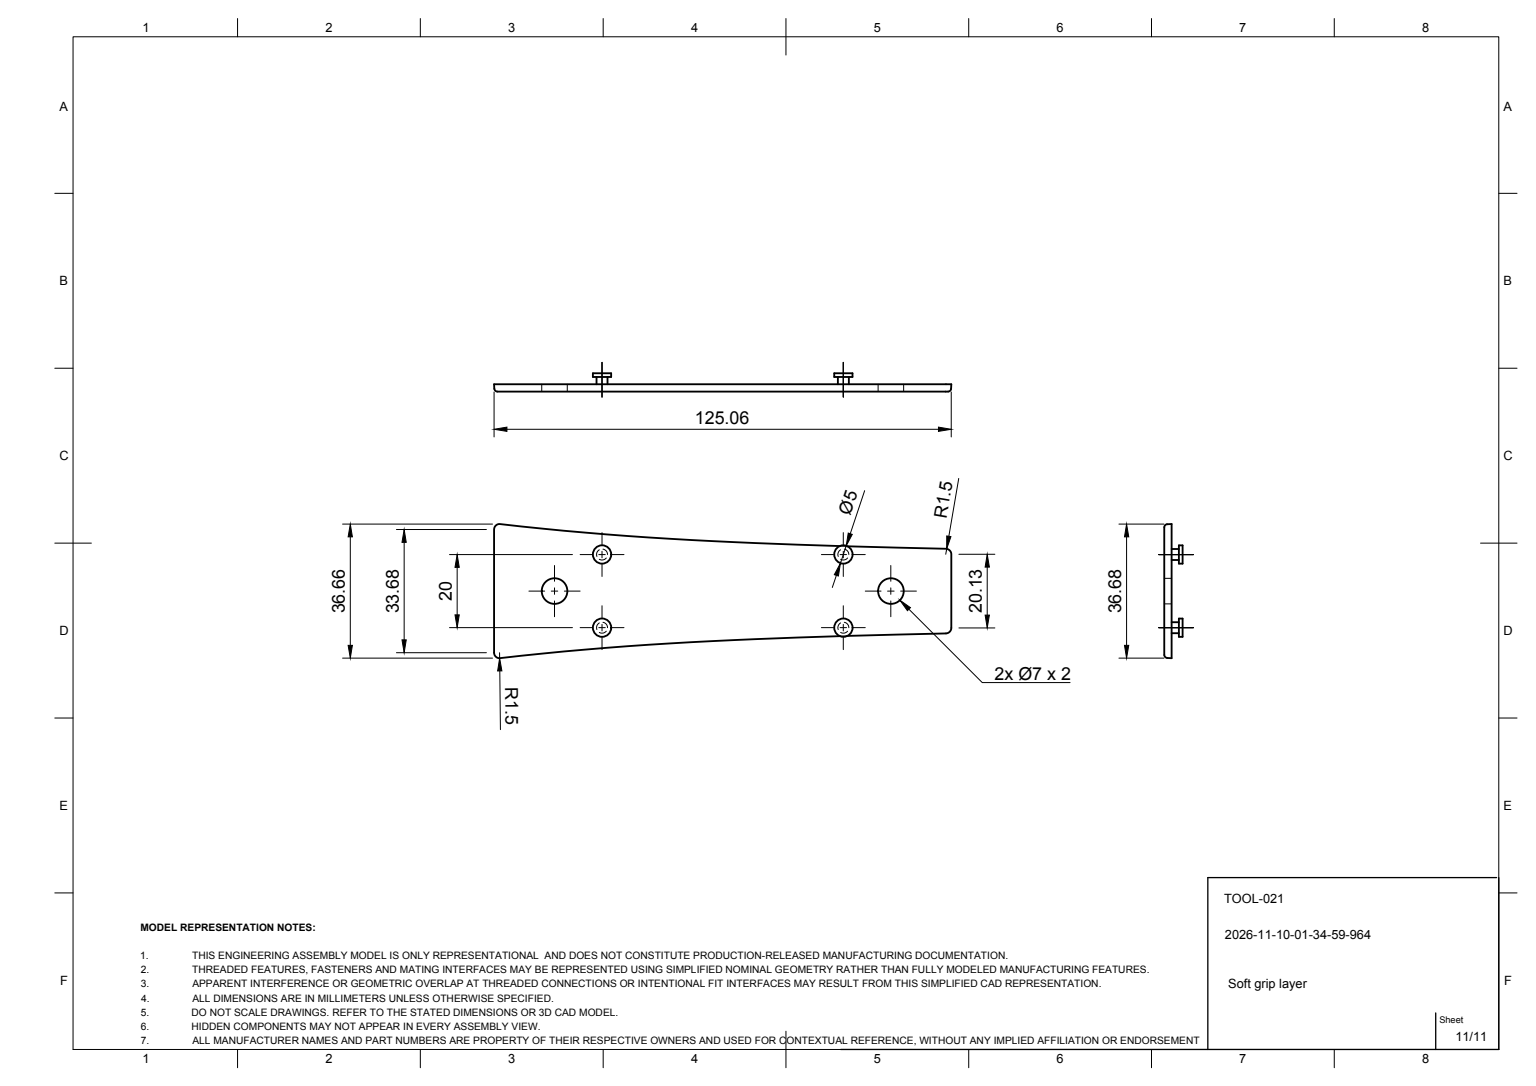
ISO-10303-21;
HEADER;
/* Generated by software containing ST-Developer
 * from STEP Tools, Inc. (www.steptools.com) 
 */

FILE_DESCRIPTION(
/* description */ (''),
/* implementation_level */ '2;1');

FILE_NAME(
/* name */ 'Soft grip layer.step',
/* time_stamp */ '2026-11-10T09:05:57-08:00',
/* author */ (''),
/* organization */ (''),
/* preprocessor_version */ 'ST-DEVELOPER v20.2',
/* originating_system */ 'Autodesk Translation Framework v15.17.0.0',
/* authorisation */ '');

FILE_SCHEMA (('AUTOMOTIVE_DESIGN { 1 0 10303 214 3 1 1 }'));
ENDSEC;

DATA;
#10=MECHANICAL_DESIGN_GEOMETRIC_PRESENTATION_REPRESENTATION('',(#571),#19618);
#155=B_SPLINE_SURFACE_WITH_KNOTS('',3,3,((#13946,#13947,#13948,#13949,#13950),
(#13951,#13952,#13953,#13954,#13955),(#13956,#13957,#13958,#13959,#13960),
(#13961,#13962,#13963,#13964,#13965),(#13966,#13967,#13968,#13969,#13970)),
 .UNSPECIFIED.,.F.,.F.,.F.,(4,1,4),(4,1,4),(0.,0.571428571428571,1.),(0.,
0.0505788685273923,0.118017359897249),.UNSPECIFIED.);
#156=B_SPLINE_SURFACE_WITH_KNOTS('',3,3,((#13993,#13994,#13995,#13996,#13997),
(#13998,#13999,#14000,#14001,#14002),(#14003,#14004,#14005,#14006,#14007),
(#14008,#14009,#14010,#14011,#14012),(#14013,#14014,#14015,#14016,#14017)),
 .UNSPECIFIED.,.F.,.F.,.F.,(4,1,4),(4,1,4),(0.,0.571428571428571,1.),(0.,
0.0505788685278266,0.118017359898262),.UNSPECIFIED.);
#157=B_SPLINE_SURFACE_WITH_KNOTS('',3,3,((#14031,#14032,#14033,#14034,#14035),
(#14036,#14037,#14038,#14039,#14040),(#14041,#14042,#14043,#14044,#14045),
(#14046,#14047,#14048,#14049,#14050),(#14051,#14052,#14053,#14054,#14055)),
 .UNSPECIFIED.,.F.,.F.,.F.,(4,1,4),(4,1,4),(0.,0.571428571428571,1.),(0.,
5.23288834931112,12.2100728150593),.UNSPECIFIED.);
#158=B_SPLINE_SURFACE_WITH_KNOTS('',3,3,((#14069,#14070,#14071,#14072,#14073),
(#14074,#14075,#14076,#14077,#14078),(#14079,#14080,#14081,#14082,#14083),
(#14084,#14085,#14086,#14087,#14088),(#14089,#14090,#14091,#14092,#14093)),
 .UNSPECIFIED.,.F.,.F.,.F.,(4,1,4),(4,1,4),(0.,0.571428571428571,1.),(1.97133828064127E-11,
0.0463413823988794,0.108129892237767),.UNSPECIFIED.);
#159=B_SPLINE_SURFACE_WITH_KNOTS('',3,3,((#14113,#14114,#14115,#14116,#14117),
(#14118,#14119,#14120,#14121,#14122),(#14123,#14124,#14125,#14126,#14127),
(#14128,#14129,#14130,#14131,#14132),(#14133,#14134,#14135,#14136,#14137)),
 .UNSPECIFIED.,.F.,.F.,.F.,(4,1,4),(4,1,4),(0.,0.571428571428571,1.),(0.,
0.0463413823743492,0.108129892206815),.UNSPECIFIED.);
#160=B_SPLINE_SURFACE_WITH_KNOTS('',3,3,((#14151,#14152,#14153,#14154,#14155),
(#14156,#14157,#14158,#14159,#14160),(#14161,#14162,#14163,#14164,#14165),
(#14166,#14167,#14168,#14169,#14170),(#14171,#14172,#14173,#14174,#14175)),
 .UNSPECIFIED.,.F.,.F.,.F.,(4,1,4),(4,1,4),(0.,0.571428571428571,1.),(6.51086303075479E-13,
6.97718480957529,12.2100734167563),.UNSPECIFIED.);
#161=B_SPLINE_SURFACE_WITH_KNOTS('',3,3,((#14198,#14199,#14200,#14201),
(#14202,#14203,#14204,#14205),(#14206,#14207,#14208,#14209),(#14210,#14211,
#14212,#14213),(#14214,#14215,#14216,#14217)),.UNSPECIFIED.,.F.,.F.,.F.,
(4,1,4),(4,4),(0.,0.571428571428571,1.),(-0.00308447593286339,0.124708996845866),
 .UNSPECIFIED.);
#162=B_SPLINE_SURFACE_WITH_KNOTS('',3,3,((#14251,#14252,#14253,#14254),
(#14255,#14256,#14257,#14258),(#14259,#14260,#14261,#14262),(#14263,#14264,
#14265,#14266)),.UNSPECIFIED.,.F.,.F.,.F.,(4,4),(4,4),(0.0116899650356219,
0.986620910196183),(0.,0.621418053543664),.UNSPECIFIED.);
#163=B_SPLINE_SURFACE_WITH_KNOTS('',3,3,((#14276,#14277,#14278,#14279),
(#14280,#14281,#14282,#14283),(#14284,#14285,#14286,#14287),(#14288,#14289,
#14290,#14291),(#14292,#14293,#14294,#14295),(#14296,#14297,#14298,#14299)),
 .UNSPECIFIED.,.F.,.F.,.F.,(4,1,1,4),(4,4),(0.,0.285714285714286,0.571428571428571,
1.),(-0.00421817271916687,0.124025126494243),.UNSPECIFIED.);
#164=B_SPLINE_SURFACE_WITH_KNOTS('',3,3,((#14347,#14348,#14349,#14350),
(#14351,#14352,#14353,#14354),(#14355,#14356,#14357,#14358),(#14359,#14360,
#14361,#14362),(#14363,#14364,#14365,#14366)),.UNSPECIFIED.,.F.,.F.,.F.,
(4,1,4),(4,4),(0.,0.571428571428571,1.),(-0.00306862226109154,0.124708996851356),
 .UNSPECIFIED.);
#165=B_SPLINE_SURFACE_WITH_KNOTS('',3,3,((#14400,#14401,#14402,#14403),
(#14404,#14405,#14406,#14407),(#14408,#14409,#14410,#14411),(#14412,#14413,
#14414,#14415),(#14416,#14417,#14418,#14419),(#14420,#14421,#14422,#14423)),
 .UNSPECIFIED.,.F.,.F.,.F.,(4,1,1,4),(4,4),(0.,0.285714285714286,0.571428571428571,
1.),(-0.00430078538920315,0.12402512649425),.UNSPECIFIED.);
#166=B_SPLINE_SURFACE_WITH_KNOTS('',3,3,((#14468,#14469,#14470,#14471),
(#14472,#14473,#14474,#14475),(#14476,#14477,#14478,#14479),(#14480,#14481,
#14482,#14483)),.UNSPECIFIED.,.F.,.F.,.F.,(4,4),(4,4),(0.0133790898038168,
0.988310034964378),(0.,0.621418053491537),.UNSPECIFIED.);
#363=B_SPLINE_CURVE_WITH_KNOTS('',3,(#13975,#13976,#13977,#13978,#13979),
 .UNSPECIFIED.,.F.,.F.,(4,1,4),(-0.118017359897249,-0.0505788685273923,
0.),.UNSPECIFIED.);
#364=B_SPLINE_CURVE_WITH_KNOTS('',3,(#13982,#13983,#13984,#13985,#13986),
 .UNSPECIFIED.,.F.,.F.,(4,1,4),(0.,0.0505788685273923,0.118017359897249),
 .UNSPECIFIED.);
#365=B_SPLINE_CURVE_WITH_KNOTS('',3,(#14021,#14022,#14023,#14024,#14025),
 .UNSPECIFIED.,.F.,.F.,(4,1,4),(-0.118017359898262,-0.0505788685278266,
0.),.UNSPECIFIED.);
#366=B_SPLINE_CURVE_WITH_KNOTS('',3,(#14026,#14027,#14028,#14029,#14030),
 .UNSPECIFIED.,.F.,.F.,(4,1,4),(0.,0.0505788685278266,0.118017359898262),
 .UNSPECIFIED.);
#367=B_SPLINE_CURVE_WITH_KNOTS('',3,(#14059,#14060,#14061,#14062,#14063),
 .UNSPECIFIED.,.F.,.F.,(4,1,4),(-12.2100728150593,-5.23288834931112,0.),
 .UNSPECIFIED.);
#368=B_SPLINE_CURVE_WITH_KNOTS('',3,(#14064,#14065,#14066,#14067,#14068),
 .UNSPECIFIED.,.F.,.F.,(4,1,4),(0.,5.23288834931112,12.2100728150593),
 .UNSPECIFIED.);
#369=B_SPLINE_CURVE_WITH_KNOTS('',3,(#14097,#14098,#14099,#14100,#14101),
 .UNSPECIFIED.,.F.,.F.,(4,1,4),(-0.108129892237767,-0.0463413823988794,
-1.97133828064127E-11),.UNSPECIFIED.);
#370=B_SPLINE_CURVE_WITH_KNOTS('',3,(#14102,#14103,#14104,#14105,#14106),
 .UNSPECIFIED.,.F.,.F.,(4,1,4),(1.97133828064127E-11,0.0463413823988794,
0.108129892237767),.UNSPECIFIED.);
#371=B_SPLINE_CURVE_WITH_KNOTS('',3,(#14141,#14142,#14143,#14144,#14145),
 .UNSPECIFIED.,.F.,.F.,(4,1,4),(-0.108129892206815,-0.0463413823743492,
0.),.UNSPECIFIED.);
#372=B_SPLINE_CURVE_WITH_KNOTS('',3,(#14146,#14147,#14148,#14149,#14150),
 .UNSPECIFIED.,.F.,.F.,(4,1,4),(0.,0.0463413823743492,0.108129892206815),
 .UNSPECIFIED.);
#373=B_SPLINE_CURVE_WITH_KNOTS('',3,(#14176,#14177,#14178,#14179,#14180),
 .UNSPECIFIED.,.F.,.F.,(4,1,4),(-12.2100734167563,-6.97718480957529,-6.51086303075479E-13),
 .UNSPECIFIED.);
#374=B_SPLINE_CURVE_WITH_KNOTS('',3,(#14181,#14182,#14183,#14184,#14185),
 .UNSPECIFIED.,.F.,.F.,(4,1,4),(6.51086303075479E-13,6.97718480957529,12.2100734167563),
 .UNSPECIFIED.);
#375=B_SPLINE_CURVE_WITH_KNOTS('',3,(#14188,#14189,#14190,#14191),
 .UNSPECIFIED.,.F.,.F.,(4,4),(0.000181689894813921,0.124708996845866),
 .UNSPECIFIED.);
#376=B_SPLINE_CURVE_WITH_KNOTS('',3,(#14194,#14195,#14196,#14197),
 .UNSPECIFIED.,.F.,.F.,(4,4),(-0.124708996851356,-0.000181689894814102),
 .UNSPECIFIED.);
#377=B_SPLINE_CURVE_WITH_KNOTS('',3,(#14219,#14220,#14221,#14222),
 .UNSPECIFIED.,.F.,.F.,(4,4),(-0.124624122980966,-1.27068494615301E-16),
 .UNSPECIFIED.);
#378=B_SPLINE_CURVE_WITH_KNOTS('',3,(#14223,#14224,#14225,#14226,#14227,
#14228,#14229,#14230,#14231,#14232,#14233,#14234,#14235,#14236,#14237,#14238,
#14239,#14240,#14241,#14242,#14243,#14244,#14245,#14246,#14247,#14248,#14249,
#14250),.UNSPECIFIED.,.F.,.F.,(4,3,3,3,3,3,3,3,3,4),(0.,0.0322747504276753,
0.0586406101183928,0.090870813631105,0.0996503787243826,0.117132790114159,
0.149546322800321,0.175583390425035,0.207787925145658,0.232457773984835),
 .UNSPECIFIED.);
#379=B_SPLINE_CURVE_WITH_KNOTS('',3,(#14268,#14269,#14270,#14271),
 .UNSPECIFIED.,.F.,.F.,(4,4),(6.28713621962651E-9,0.124025126494243),
 .UNSPECIFIED.);
#380=B_SPLINE_CURVE_WITH_KNOTS('',3,(#14272,#14273,#14274,#14275),
 .UNSPECIFIED.,.F.,.F.,(4,4),(0.0116899650356219,0.986620910196183),
 .UNSPECIFIED.);
#381=B_SPLINE_CURVE_WITH_KNOTS('',3,(#14301,#14302,#14303,#14304),
 .UNSPECIFIED.,.F.,.F.,(4,4),(-0.12358375933533,0.000944809985246663),
 .UNSPECIFIED.);
#382=B_SPLINE_CURVE_WITH_KNOTS('',3,(#14305,#14306,#14307,#14308,#14309,
#14310,#14311,#14312,#14313,#14314,#14315,#14316,#14317,#14318,#14319,#14320,
#14321,#14322,#14323,#14324,#14325,#14326,#14327,#14328,#14329,#14330,#14331,
#14332,#14333,#14334,#14335,#14336,#14337,#14338),.UNSPECIFIED.,.F.,.F.,
(4,3,3,3,3,3,3,3,3,3,3,4),(0.,0.0322568536241053,0.0586526138523664,0.0909514856947606,
0.108742407475907,0.117151788463556,0.149394351344039,0.175600627102286,
0.181167420983902,0.214570374458228,0.246736309066329,0.253563811229603),
 .UNSPECIFIED.);
#383=B_SPLINE_CURVE_WITH_KNOTS('',3,(#14342,#14343,#14344,#14345),
 .UNSPECIFIED.,.F.,.F.,(4,4),(-0.000944809985246617,0.123583759335329),
 .UNSPECIFIED.);
#384=B_SPLINE_CURVE_WITH_KNOTS('',3,(#14368,#14369,#14370,#14371,#14372,
#14373,#14374,#14375,#14376,#14377,#14378,#14379,#14380,#14381,#14382,#14383,
#14384,#14385,#14386,#14387,#14388,#14389,#14390,#14391,#14392,#14393,#14394,
#14395),.UNSPECIFIED.,.F.,.F.,(4,3,3,3,3,3,3,3,3,4),(0.,0.0322765438584903,
0.0586513922310012,0.0908809480268686,0.099655003871439,0.117150238497558,
0.149564657711791,0.175599638586681,0.20780211537115,0.232458396023953),
 .UNSPECIFIED.);
#385=B_SPLINE_CURVE_WITH_KNOTS('',3,(#14396,#14397,#14398,#14399),
 .UNSPECIFIED.,.F.,.F.,(4,4),(3.30031141304588E-16,0.124624122970512),
 .UNSPECIFIED.);
#386=B_SPLINE_CURVE_WITH_KNOTS('',3,(#14425,#14426,#14427,#14428),
 .UNSPECIFIED.,.F.,.F.,(4,4),(-0.12402512649425,-6.28713634712869E-9),
 .UNSPECIFIED.);
#387=B_SPLINE_CURVE_WITH_KNOTS('',3,(#14429,#14430,#14431,#14432,#14433,
#14434,#14435,#14436,#14437,#14438,#14439,#14440,#14441,#14442,#14443,#14444,
#14445,#14446,#14447,#14448,#14449,#14450,#14451,#14452,#14453,#14454,#14455,
#14456,#14457,#14458,#14459,#14460,#14461,#14462),.UNSPECIFIED.,.F.,.F.,
(4,3,3,3,3,3,3,3,3,3,3,4),(0.,0.0322666769662355,0.0587055335553437,0.0910029078093924,
0.108768157423115,0.117242626226166,0.149488313345073,0.175692943342501,
0.181189289804584,0.214619150478997,0.24677571115805,0.253566775541772),
 .UNSPECIFIED.);
#388=B_SPLINE_CURVE_WITH_KNOTS('',3,(#14464,#14465,#14466,#14467),
 .UNSPECIFIED.,.F.,.F.,(4,4),(0.0133790898038168,0.988310034964378),
 .UNSPECIFIED.);
#551=SHAPE_REPRESENTATION_RELATIONSHIP('SRR','None',#19671,#561);
#561=ADVANCED_BREP_SHAPE_REPRESENTATION('',(#581),#19614);
#571=STYLED_ITEM('',(#19732),#581);
#581=MANIFOLD_SOLID_BREP('Body1',#7109);
#642=FACE_BOUND('',#1545,.T.);
#643=FACE_BOUND('',#1549,.T.);
#644=FACE_BOUND('',#1553,.T.);
#645=FACE_BOUND('',#1557,.T.);
#646=FACE_BOUND('',#1577,.T.);
#647=FACE_BOUND('',#1578,.T.);
#648=FACE_BOUND('',#1583,.T.);
#649=FACE_BOUND('',#1584,.T.);
#650=FACE_BOUND('',#1585,.T.);
#651=FACE_BOUND('',#1586,.T.);
#652=FACE_BOUND('',#1587,.T.);
#653=FACE_BOUND('',#1588,.T.);
#789=PLANE('',#7590);
#790=PLANE('',#7595);
#791=PLANE('',#7596);
#792=PLANE('',#7601);
#793=PLANE('',#7602);
#794=PLANE('',#7607);
#795=PLANE('',#7608);
#796=PLANE('',#7613);
#797=PLANE('',#7632);
#798=PLANE('',#7633);
#799=PLANE('',#7634);
#800=PLANE('',#7635);
#1086=FACE_OUTER_BOUND('',#1542,.T.);
#1087=FACE_OUTER_BOUND('',#1543,.T.);
#1088=FACE_OUTER_BOUND('',#1544,.T.);
#1089=FACE_OUTER_BOUND('',#1546,.T.);
#1090=FACE_OUTER_BOUND('',#1547,.T.);
#1091=FACE_OUTER_BOUND('',#1548,.T.);
#1092=FACE_OUTER_BOUND('',#1550,.T.);
#1093=FACE_OUTER_BOUND('',#1551,.T.);
#1094=FACE_OUTER_BOUND('',#1552,.T.);
#1095=FACE_OUTER_BOUND('',#1554,.T.);
#1096=FACE_OUTER_BOUND('',#1555,.T.);
#1097=FACE_OUTER_BOUND('',#1556,.T.);
#1098=FACE_OUTER_BOUND('',#1558,.T.);
#1099=FACE_OUTER_BOUND('',#1559,.T.);
#1100=FACE_OUTER_BOUND('',#1560,.T.);
#1101=FACE_OUTER_BOUND('',#1561,.T.);
#1102=FACE_OUTER_BOUND('',#1562,.T.);
#1103=FACE_OUTER_BOUND('',#1563,.T.);
#1104=FACE_OUTER_BOUND('',#1564,.T.);
#1105=FACE_OUTER_BOUND('',#1565,.T.);
#1106=FACE_OUTER_BOUND('',#1566,.T.);
#1107=FACE_OUTER_BOUND('',#1567,.T.);
#1108=FACE_OUTER_BOUND('',#1568,.T.);
#1109=FACE_OUTER_BOUND('',#1569,.T.);
#1110=FACE_OUTER_BOUND('',#1570,.T.);
#1111=FACE_OUTER_BOUND('',#1571,.T.);
#1112=FACE_OUTER_BOUND('',#1572,.T.);
#1113=FACE_OUTER_BOUND('',#1573,.T.);
#1114=FACE_OUTER_BOUND('',#1574,.T.);
#1115=FACE_OUTER_BOUND('',#1575,.T.);
#1116=FACE_OUTER_BOUND('',#1576,.T.);
#1117=FACE_OUTER_BOUND('',#1579,.T.);
#1118=FACE_OUTER_BOUND('',#1580,.T.);
#1119=FACE_OUTER_BOUND('',#1581,.T.);
#1120=FACE_OUTER_BOUND('',#1582,.T.);
#1121=FACE_OUTER_BOUND('',#1589,.T.);
#1542=EDGE_LOOP('',(#5854,#5855,#5856,#5857));
#1543=EDGE_LOOP('',(#5858,#5859,#5860,#5861));
#1544=EDGE_LOOP('',(#5862));
#1545=EDGE_LOOP('',(#5863));
#1546=EDGE_LOOP('',(#5864,#5865,#5866,#5867));
#1547=EDGE_LOOP('',(#5868));
#1548=EDGE_LOOP('',(#5869));
#1549=EDGE_LOOP('',(#5870));
#1550=EDGE_LOOP('',(#5871,#5872,#5873,#5874));
#1551=EDGE_LOOP('',(#5875));
#1552=EDGE_LOOP('',(#5876));
#1553=EDGE_LOOP('',(#5877));
#1554=EDGE_LOOP('',(#5878,#5879,#5880,#5881));
#1555=EDGE_LOOP('',(#5882));
#1556=EDGE_LOOP('',(#5883));
#1557=EDGE_LOOP('',(#5884));
#1558=EDGE_LOOP('',(#5885,#5886,#5887,#5888));
#1559=EDGE_LOOP('',(#5889));
#1560=EDGE_LOOP('',(#5890,#5891,#5892,#5893));
#1561=EDGE_LOOP('',(#5894,#5895,#5896,#5897));
#1562=EDGE_LOOP('',(#5898,#5899,#5900,#5901));
#1563=EDGE_LOOP('',(#5902,#5903,#5904,#5905));
#1564=EDGE_LOOP('',(#5906,#5907,#5908,#5909));
#1565=EDGE_LOOP('',(#5910,#5911,#5912,#5913));
#1566=EDGE_LOOP('',(#5914,#5915,#5916,#5917));
#1567=EDGE_LOOP('',(#5918,#5919,#5920,#5921));
#1568=EDGE_LOOP('',(#5922,#5923,#5924,#5925));
#1569=EDGE_LOOP('',(#5926,#5927,#5928,#5929));
#1570=EDGE_LOOP('',(#5930,#5931,#5932,#5933));
#1571=EDGE_LOOP('',(#5934,#5935,#5936,#5937));
#1572=EDGE_LOOP('',(#5938,#5939,#5940,#5941));
#1573=EDGE_LOOP('',(#5942,#5943,#5944,#5945));
#1574=EDGE_LOOP('',(#5946,#5947,#5948,#5949));
#1575=EDGE_LOOP('',(#5950,#5951,#5952,#5953));
#1576=EDGE_LOOP('',(#5954,#5955,#5956,#5957,#5958,#5959,#5960,#5961));
#1577=EDGE_LOOP('',(#5962));
#1578=EDGE_LOOP('',(#5963));
#1579=EDGE_LOOP('',(#5964,#5965,#5966,#5967));
#1580=EDGE_LOOP('',(#5968,#5969,#5970,#5971));
#1581=EDGE_LOOP('',(#5972,#5973,#5974,#5975));
#1582=EDGE_LOOP('',(#5976,#5977,#5978,#5979,#5980,#5981,#5982,#5983));
#1583=EDGE_LOOP('',(#5984));
#1584=EDGE_LOOP('',(#5985));
#1585=EDGE_LOOP('',(#5986));
#1586=EDGE_LOOP('',(#5987));
#1587=EDGE_LOOP('',(#5988));
#1588=EDGE_LOOP('',(#5989));
#1589=EDGE_LOOP('',(#5990,#5991,#5992,#5993));
#2031=LINE('',#13882,#2490);
#2032=LINE('',#13888,#2491);
#2033=LINE('',#13898,#2492);
#2034=LINE('',#13908,#2493);
#2035=LINE('',#13918,#2494);
#2036=LINE('',#13928,#2495);
#2037=LINE('',#13932,#2496);
#2038=LINE('',#13936,#2497);
#2039=LINE('',#13940,#2498);
#2040=LINE('',#13944,#2499);
#2041=LINE('',#13991,#2500);
#2042=LINE('',#13992,#2501);
#2043=LINE('',#14111,#2502);
#2044=LINE('',#14112,#2503);
#2045=LINE('',#14193,#2504);
#2046=LINE('',#14346,#2505);
#2490=VECTOR('',#8826,0.35);
#2491=VECTOR('',#8833,0.35);
#2492=VECTOR('',#8846,0.25);
#2493=VECTOR('',#8859,0.25);
#2494=VECTOR('',#8872,0.25);
#2495=VECTOR('',#8885,0.25);
#2496=VECTOR('',#8890,0.15);
#2497=VECTOR('',#8895,0.15);
#2498=VECTOR('',#8900,0.15);
#2499=VECTOR('',#8905,0.15);
#2500=VECTOR('',#8916,1.);
#2501=VECTOR('',#8917,1.);
#2502=VECTOR('',#8928,1.);
#2503=VECTOR('',#8929,1.);
#2504=VECTOR('',#8934,1.);
#2505=VECTOR('',#8939,1.);
#2766=CIRCLE('',#7585,0.35);
#2767=CIRCLE('',#7586,0.35);
#2768=CIRCLE('',#7588,0.35);
#2769=CIRCLE('',#7589,0.35);
#2770=CIRCLE('',#7591,0.25);
#2771=CIRCLE('',#7592,0.15);
#2772=CIRCLE('',#7594,0.25);
#2773=CIRCLE('',#7597,0.25);
#2774=CIRCLE('',#7598,0.15);
#2775=CIRCLE('',#7600,0.25);
#2776=CIRCLE('',#7603,0.25);
#2777=CIRCLE('',#7604,0.15);
#2778=CIRCLE('',#7606,0.25);
#2779=CIRCLE('',#7609,0.25);
#2780=CIRCLE('',#7610,0.15);
#2781=CIRCLE('',#7612,0.25);
#2782=CIRCLE('',#7615,0.15);
#2783=CIRCLE('',#7617,0.15);
#2784=CIRCLE('',#7619,0.15);
#2785=CIRCLE('',#7621,0.15);
#2786=CIRCLE('',#7622,0.0800000000000001);
#2787=CIRCLE('',#7623,0.0800000000000001);
#2788=CIRCLE('',#7625,0.0800000000000001);
#2789=CIRCLE('',#7626,0.0800000000000001);
#2790=CIRCLE('',#7627,0.0800000000000001);
#2791=CIRCLE('',#7628,0.0800000000000003);
#2792=CIRCLE('',#7630,0.0800000000000001);
#2793=CIRCLE('',#7631,0.0800000000000003);
#3245=VERTEX_POINT('',#13879);
#3246=VERTEX_POINT('',#13881);
#3247=VERTEX_POINT('',#13885);
#3248=VERTEX_POINT('',#13887);
#3249=VERTEX_POINT('',#13891);
#3250=VERTEX_POINT('',#13893);
#3251=VERTEX_POINT('',#13896);
#3252=VERTEX_POINT('',#13901);
#3253=VERTEX_POINT('',#13903);
#3254=VERTEX_POINT('',#13906);
#3255=VERTEX_POINT('',#13911);
#3256=VERTEX_POINT('',#13913);
#3257=VERTEX_POINT('',#13916);
#3258=VERTEX_POINT('',#13921);
#3259=VERTEX_POINT('',#13923);
#3260=VERTEX_POINT('',#13926);
#3261=VERTEX_POINT('',#13931);
#3262=VERTEX_POINT('',#13935);
#3263=VERTEX_POINT('',#13939);
#3264=VERTEX_POINT('',#13943);
#3265=VERTEX_POINT('',#13971);
#3266=VERTEX_POINT('',#13972);
#3267=VERTEX_POINT('',#13974);
#3268=VERTEX_POINT('',#13980);
#3269=VERTEX_POINT('',#13988);
#3270=VERTEX_POINT('',#13989);
#3271=VERTEX_POINT('',#14018);
#3272=VERTEX_POINT('',#14019);
#3273=VERTEX_POINT('',#14056);
#3274=VERTEX_POINT('',#14057);
#3275=VERTEX_POINT('',#14094);
#3276=VERTEX_POINT('',#14095);
#3277=VERTEX_POINT('',#14108);
#3278=VERTEX_POINT('',#14109);
#3279=VERTEX_POINT('',#14138);
#3280=VERTEX_POINT('',#14139);
#3281=VERTEX_POINT('',#14187);
#3282=VERTEX_POINT('',#14192);
#3283=VERTEX_POINT('',#14218);
#3284=VERTEX_POINT('',#14267);
#3285=VERTEX_POINT('',#14300);
#3286=VERTEX_POINT('',#14341);
#3287=VERTEX_POINT('',#14367);
#3288=VERTEX_POINT('',#14424);
#4152=EDGE_CURVE('',#3245,#3245,#2766,.T.);
#4153=EDGE_CURVE('',#3245,#3246,#2031,.T.);
#4154=EDGE_CURVE('',#3246,#3246,#2767,.T.);
#4155=EDGE_CURVE('',#3247,#3247,#2768,.T.);
#4156=EDGE_CURVE('',#3247,#3248,#2032,.T.);
#4157=EDGE_CURVE('',#3248,#3248,#2769,.T.);
#4158=EDGE_CURVE('',#3249,#3249,#2770,.T.);
#4159=EDGE_CURVE('',#3250,#3250,#2771,.T.);
#4160=EDGE_CURVE('',#3251,#3251,#2772,.T.);
#4161=EDGE_CURVE('',#3251,#3249,#2033,.T.);
#4162=EDGE_CURVE('',#3252,#3252,#2773,.T.);
#4163=EDGE_CURVE('',#3253,#3253,#2774,.T.);
#4164=EDGE_CURVE('',#3254,#3254,#2775,.T.);
#4165=EDGE_CURVE('',#3254,#3252,#2034,.T.);
#4166=EDGE_CURVE('',#3255,#3255,#2776,.T.);
#4167=EDGE_CURVE('',#3256,#3256,#2777,.T.);
#4168=EDGE_CURVE('',#3257,#3257,#2778,.T.);
#4169=EDGE_CURVE('',#3257,#3255,#2035,.T.);
#4170=EDGE_CURVE('',#3258,#3258,#2779,.T.);
#4171=EDGE_CURVE('',#3259,#3259,#2780,.T.);
#4172=EDGE_CURVE('',#3260,#3260,#2781,.T.);
#4173=EDGE_CURVE('',#3260,#3258,#2036,.T.);
#4174=EDGE_CURVE('',#3250,#3261,#2037,.T.);
#4175=EDGE_CURVE('',#3261,#3261,#2782,.T.);
#4176=EDGE_CURVE('',#3253,#3262,#2038,.T.);
#4177=EDGE_CURVE('',#3262,#3262,#2783,.T.);
#4178=EDGE_CURVE('',#3256,#3263,#2039,.T.);
#4179=EDGE_CURVE('',#3263,#3263,#2784,.T.);
#4180=EDGE_CURVE('',#3259,#3264,#2040,.T.);
#4181=EDGE_CURVE('',#3264,#3264,#2785,.T.);
#4182=EDGE_CURVE('',#3265,#3266,#2786,.T.);
#4183=EDGE_CURVE('',#3266,#3267,#363,.T.);
#4184=EDGE_CURVE('',#3267,#3268,#2787,.T.);
#4185=EDGE_CURVE('',#3268,#3265,#364,.T.);
#4186=EDGE_CURVE('',#3269,#3270,#2788,.T.);
#4187=EDGE_CURVE('',#3270,#3266,#2041,.T.);
#4188=EDGE_CURVE('',#3265,#3269,#2042,.T.);
#4189=EDGE_CURVE('',#3271,#3272,#2789,.T.);
#4190=EDGE_CURVE('',#3272,#3270,#365,.T.);
#4191=EDGE_CURVE('',#3269,#3271,#366,.T.);
#4192=EDGE_CURVE('',#3273,#3274,#2790,.T.);
#4193=EDGE_CURVE('',#3274,#3272,#367,.T.);
#4194=EDGE_CURVE('',#3271,#3273,#368,.T.);
#4195=EDGE_CURVE('',#3275,#3276,#2791,.T.);
#4196=EDGE_CURVE('',#3276,#3274,#369,.T.);
#4197=EDGE_CURVE('',#3273,#3275,#370,.T.);
#4198=EDGE_CURVE('',#3277,#3278,#2792,.T.);
#4199=EDGE_CURVE('',#3278,#3276,#2043,.T.);
#4200=EDGE_CURVE('',#3275,#3277,#2044,.T.);
#4201=EDGE_CURVE('',#3279,#3280,#2793,.T.);
#4202=EDGE_CURVE('',#3280,#3278,#371,.T.);
#4203=EDGE_CURVE('',#3277,#3279,#372,.T.);
#4204=EDGE_CURVE('',#3267,#3280,#373,.T.);
#4205=EDGE_CURVE('',#3279,#3268,#374,.T.);
#4206=EDGE_CURVE('',#3281,#3278,#375,.T.);
#4207=EDGE_CURVE('',#3282,#3281,#2045,.T.);
#4208=EDGE_CURVE('',#3276,#3282,#376,.T.);
#4209=EDGE_CURVE('',#3280,#3283,#377,.T.);
#4210=EDGE_CURVE('',#3283,#3281,#378,.T.);
#4211=EDGE_CURVE('',#3284,#3267,#379,.T.);
#4212=EDGE_CURVE('',#3283,#3284,#380,.T.);
#4213=EDGE_CURVE('',#3266,#3285,#381,.T.);
#4214=EDGE_CURVE('',#3285,#3284,#382,.T.);
#4215=EDGE_CURVE('',#3286,#3270,#383,.T.);
#4216=EDGE_CURVE('',#3285,#3286,#2046,.T.);
#4217=EDGE_CURVE('',#3282,#3287,#384,.T.);
#4218=EDGE_CURVE('',#3287,#3274,#385,.T.);
#4219=EDGE_CURVE('',#3272,#3288,#386,.T.);
#4220=EDGE_CURVE('',#3288,#3286,#387,.T.);
#4221=EDGE_CURVE('',#3288,#3287,#388,.T.);
#5854=ORIENTED_EDGE('',*,*,#4152,.F.);
#5855=ORIENTED_EDGE('',*,*,#4153,.T.);
#5856=ORIENTED_EDGE('',*,*,#4154,.F.);
#5857=ORIENTED_EDGE('',*,*,#4153,.F.);
#5858=ORIENTED_EDGE('',*,*,#4155,.F.);
#5859=ORIENTED_EDGE('',*,*,#4156,.T.);
#5860=ORIENTED_EDGE('',*,*,#4157,.F.);
#5861=ORIENTED_EDGE('',*,*,#4156,.F.);
#5862=ORIENTED_EDGE('',*,*,#4158,.T.);
#5863=ORIENTED_EDGE('',*,*,#4159,.T.);
#5864=ORIENTED_EDGE('',*,*,#4160,.F.);
#5865=ORIENTED_EDGE('',*,*,#4161,.T.);
#5866=ORIENTED_EDGE('',*,*,#4158,.F.);
#5867=ORIENTED_EDGE('',*,*,#4161,.F.);
#5868=ORIENTED_EDGE('',*,*,#4160,.T.);
#5869=ORIENTED_EDGE('',*,*,#4162,.T.);
#5870=ORIENTED_EDGE('',*,*,#4163,.T.);
#5871=ORIENTED_EDGE('',*,*,#4164,.F.);
#5872=ORIENTED_EDGE('',*,*,#4165,.T.);
#5873=ORIENTED_EDGE('',*,*,#4162,.F.);
#5874=ORIENTED_EDGE('',*,*,#4165,.F.);
#5875=ORIENTED_EDGE('',*,*,#4164,.T.);
#5876=ORIENTED_EDGE('',*,*,#4166,.T.);
#5877=ORIENTED_EDGE('',*,*,#4167,.T.);
#5878=ORIENTED_EDGE('',*,*,#4168,.F.);
#5879=ORIENTED_EDGE('',*,*,#4169,.T.);
#5880=ORIENTED_EDGE('',*,*,#4166,.F.);
#5881=ORIENTED_EDGE('',*,*,#4169,.F.);
#5882=ORIENTED_EDGE('',*,*,#4168,.T.);
#5883=ORIENTED_EDGE('',*,*,#4170,.T.);
#5884=ORIENTED_EDGE('',*,*,#4171,.T.);
#5885=ORIENTED_EDGE('',*,*,#4172,.F.);
#5886=ORIENTED_EDGE('',*,*,#4173,.T.);
#5887=ORIENTED_EDGE('',*,*,#4170,.F.);
#5888=ORIENTED_EDGE('',*,*,#4173,.F.);
#5889=ORIENTED_EDGE('',*,*,#4172,.T.);
#5890=ORIENTED_EDGE('',*,*,#4159,.F.);
#5891=ORIENTED_EDGE('',*,*,#4174,.T.);
#5892=ORIENTED_EDGE('',*,*,#4175,.F.);
#5893=ORIENTED_EDGE('',*,*,#4174,.F.);
#5894=ORIENTED_EDGE('',*,*,#4163,.F.);
#5895=ORIENTED_EDGE('',*,*,#4176,.T.);
#5896=ORIENTED_EDGE('',*,*,#4177,.F.);
#5897=ORIENTED_EDGE('',*,*,#4176,.F.);
#5898=ORIENTED_EDGE('',*,*,#4167,.F.);
#5899=ORIENTED_EDGE('',*,*,#4178,.T.);
#5900=ORIENTED_EDGE('',*,*,#4179,.F.);
#5901=ORIENTED_EDGE('',*,*,#4178,.F.);
#5902=ORIENTED_EDGE('',*,*,#4171,.F.);
#5903=ORIENTED_EDGE('',*,*,#4180,.T.);
#5904=ORIENTED_EDGE('',*,*,#4181,.F.);
#5905=ORIENTED_EDGE('',*,*,#4180,.F.);
#5906=ORIENTED_EDGE('',*,*,#4182,.T.);
#5907=ORIENTED_EDGE('',*,*,#4183,.T.);
#5908=ORIENTED_EDGE('',*,*,#4184,.T.);
#5909=ORIENTED_EDGE('',*,*,#4185,.T.);
#5910=ORIENTED_EDGE('',*,*,#4186,.T.);
#5911=ORIENTED_EDGE('',*,*,#4187,.T.);
#5912=ORIENTED_EDGE('',*,*,#4182,.F.);
#5913=ORIENTED_EDGE('',*,*,#4188,.T.);
#5914=ORIENTED_EDGE('',*,*,#4189,.T.);
#5915=ORIENTED_EDGE('',*,*,#4190,.T.);
#5916=ORIENTED_EDGE('',*,*,#4186,.F.);
#5917=ORIENTED_EDGE('',*,*,#4191,.T.);
#5918=ORIENTED_EDGE('',*,*,#4192,.T.);
#5919=ORIENTED_EDGE('',*,*,#4193,.T.);
#5920=ORIENTED_EDGE('',*,*,#4189,.F.);
#5921=ORIENTED_EDGE('',*,*,#4194,.T.);
#5922=ORIENTED_EDGE('',*,*,#4195,.T.);
#5923=ORIENTED_EDGE('',*,*,#4196,.T.);
#5924=ORIENTED_EDGE('',*,*,#4192,.F.);
#5925=ORIENTED_EDGE('',*,*,#4197,.T.);
#5926=ORIENTED_EDGE('',*,*,#4198,.T.);
#5927=ORIENTED_EDGE('',*,*,#4199,.T.);
#5928=ORIENTED_EDGE('',*,*,#4195,.F.);
#5929=ORIENTED_EDGE('',*,*,#4200,.T.);
#5930=ORIENTED_EDGE('',*,*,#4201,.T.);
#5931=ORIENTED_EDGE('',*,*,#4202,.T.);
#5932=ORIENTED_EDGE('',*,*,#4198,.F.);
#5933=ORIENTED_EDGE('',*,*,#4203,.T.);
#5934=ORIENTED_EDGE('',*,*,#4184,.F.);
#5935=ORIENTED_EDGE('',*,*,#4204,.T.);
#5936=ORIENTED_EDGE('',*,*,#4201,.F.);
#5937=ORIENTED_EDGE('',*,*,#4205,.T.);
#5938=ORIENTED_EDGE('',*,*,#4199,.F.);
#5939=ORIENTED_EDGE('',*,*,#4206,.F.);
#5940=ORIENTED_EDGE('',*,*,#4207,.F.);
#5941=ORIENTED_EDGE('',*,*,#4208,.F.);
#5942=ORIENTED_EDGE('',*,*,#4202,.F.);
#5943=ORIENTED_EDGE('',*,*,#4209,.T.);
#5944=ORIENTED_EDGE('',*,*,#4210,.T.);
#5945=ORIENTED_EDGE('',*,*,#4206,.T.);
#5946=ORIENTED_EDGE('',*,*,#4204,.F.);
#5947=ORIENTED_EDGE('',*,*,#4211,.F.);
#5948=ORIENTED_EDGE('',*,*,#4212,.F.);
#5949=ORIENTED_EDGE('',*,*,#4209,.F.);
#5950=ORIENTED_EDGE('',*,*,#4183,.F.);
#5951=ORIENTED_EDGE('',*,*,#4213,.T.);
#5952=ORIENTED_EDGE('',*,*,#4214,.T.);
#5953=ORIENTED_EDGE('',*,*,#4211,.T.);
#5954=ORIENTED_EDGE('',*,*,#4185,.F.);
#5955=ORIENTED_EDGE('',*,*,#4205,.F.);
#5956=ORIENTED_EDGE('',*,*,#4203,.F.);
#5957=ORIENTED_EDGE('',*,*,#4200,.F.);
#5958=ORIENTED_EDGE('',*,*,#4197,.F.);
#5959=ORIENTED_EDGE('',*,*,#4194,.F.);
#5960=ORIENTED_EDGE('',*,*,#4191,.F.);
#5961=ORIENTED_EDGE('',*,*,#4188,.F.);
#5962=ORIENTED_EDGE('',*,*,#4152,.T.);
#5963=ORIENTED_EDGE('',*,*,#4155,.T.);
#5964=ORIENTED_EDGE('',*,*,#4187,.F.);
#5965=ORIENTED_EDGE('',*,*,#4215,.F.);
#5966=ORIENTED_EDGE('',*,*,#4216,.F.);
#5967=ORIENTED_EDGE('',*,*,#4213,.F.);
#5968=ORIENTED_EDGE('',*,*,#4196,.F.);
#5969=ORIENTED_EDGE('',*,*,#4208,.T.);
#5970=ORIENTED_EDGE('',*,*,#4217,.T.);
#5971=ORIENTED_EDGE('',*,*,#4218,.T.);
#5972=ORIENTED_EDGE('',*,*,#4190,.F.);
#5973=ORIENTED_EDGE('',*,*,#4219,.T.);
#5974=ORIENTED_EDGE('',*,*,#4220,.T.);
#5975=ORIENTED_EDGE('',*,*,#4215,.T.);
#5976=ORIENTED_EDGE('',*,*,#4214,.F.);
#5977=ORIENTED_EDGE('',*,*,#4216,.T.);
#5978=ORIENTED_EDGE('',*,*,#4220,.F.);
#5979=ORIENTED_EDGE('',*,*,#4221,.T.);
#5980=ORIENTED_EDGE('',*,*,#4217,.F.);
#5981=ORIENTED_EDGE('',*,*,#4207,.T.);
#5982=ORIENTED_EDGE('',*,*,#4210,.F.);
#5983=ORIENTED_EDGE('',*,*,#4212,.T.);
#5984=ORIENTED_EDGE('',*,*,#4154,.T.);
#5985=ORIENTED_EDGE('',*,*,#4157,.T.);
#5986=ORIENTED_EDGE('',*,*,#4175,.T.);
#5987=ORIENTED_EDGE('',*,*,#4177,.T.);
#5988=ORIENTED_EDGE('',*,*,#4179,.T.);
#5989=ORIENTED_EDGE('',*,*,#4181,.T.);
#5990=ORIENTED_EDGE('',*,*,#4193,.F.);
#5991=ORIENTED_EDGE('',*,*,#4218,.F.);
#5992=ORIENTED_EDGE('',*,*,#4221,.F.);
#5993=ORIENTED_EDGE('',*,*,#4219,.F.);
#6611=CYLINDRICAL_SURFACE('',#7584,0.35);
#6612=CYLINDRICAL_SURFACE('',#7587,0.35);
#6613=CYLINDRICAL_SURFACE('',#7593,0.25);
#6614=CYLINDRICAL_SURFACE('',#7599,0.25);
#6615=CYLINDRICAL_SURFACE('',#7605,0.25);
#6616=CYLINDRICAL_SURFACE('',#7611,0.25);
#6617=CYLINDRICAL_SURFACE('',#7614,0.15);
#6618=CYLINDRICAL_SURFACE('',#7616,0.15);
#6619=CYLINDRICAL_SURFACE('',#7618,0.15);
#6620=CYLINDRICAL_SURFACE('',#7620,0.15);
#6621=CYLINDRICAL_SURFACE('',#7624,0.08);
#6622=CYLINDRICAL_SURFACE('',#7629,0.08);
#6965=ADVANCED_FACE('',(#1086),#6611,.F.);
#6966=ADVANCED_FACE('',(#1087),#6612,.F.);
#6967=ADVANCED_FACE('',(#1088,#642),#789,.T.);
#6968=ADVANCED_FACE('',(#1089),#6613,.T.);
#6969=ADVANCED_FACE('',(#1090),#790,.F.);
#6970=ADVANCED_FACE('',(#1091,#643),#791,.T.);
#6971=ADVANCED_FACE('',(#1092),#6614,.T.);
#6972=ADVANCED_FACE('',(#1093),#792,.F.);
#6973=ADVANCED_FACE('',(#1094,#644),#793,.T.);
#6974=ADVANCED_FACE('',(#1095),#6615,.T.);
#6975=ADVANCED_FACE('',(#1096),#794,.F.);
#6976=ADVANCED_FACE('',(#1097,#645),#795,.T.);
#6977=ADVANCED_FACE('',(#1098),#6616,.T.);
#6978=ADVANCED_FACE('',(#1099),#796,.F.);
#6979=ADVANCED_FACE('',(#1100),#6617,.T.);
#6980=ADVANCED_FACE('',(#1101),#6618,.T.);
#6981=ADVANCED_FACE('',(#1102),#6619,.T.);
#6982=ADVANCED_FACE('',(#1103),#6620,.T.);
#6983=ADVANCED_FACE('',(#1104),#155,.F.);
#6984=ADVANCED_FACE('',(#1105),#6621,.T.);
#6985=ADVANCED_FACE('',(#1106),#156,.F.);
#6986=ADVANCED_FACE('',(#1107),#157,.F.);
#6987=ADVANCED_FACE('',(#1108),#158,.F.);
#6988=ADVANCED_FACE('',(#1109),#6622,.T.);
#6989=ADVANCED_FACE('',(#1110),#159,.F.);
#6990=ADVANCED_FACE('',(#1111),#160,.F.);
#6991=ADVANCED_FACE('',(#1112),#797,.F.);
#6992=ADVANCED_FACE('',(#1113),#161,.F.);
#6993=ADVANCED_FACE('',(#1114),#162,.F.);
#6994=ADVANCED_FACE('',(#1115),#163,.F.);
#6995=ADVANCED_FACE('',(#1116,#646,#647),#798,.T.);
#6996=ADVANCED_FACE('',(#1117),#799,.F.);
#6997=ADVANCED_FACE('',(#1118),#164,.F.);
#6998=ADVANCED_FACE('',(#1119),#165,.F.);
#6999=ADVANCED_FACE('',(#1120,#648,#649,#650,#651,#652,#653),#800,.F.);
#7000=ADVANCED_FACE('',(#1121),#166,.F.);
#7109=CLOSED_SHELL('',(#6965,#6966,#6967,#6968,#6969,#6970,#6971,#6972,
#6973,#6974,#6975,#6976,#6977,#6978,#6979,#6980,#6981,#6982,#6983,#6984,
#6985,#6986,#6987,#6988,#6989,#6990,#6991,#6992,#6993,#6994,#6995,#6996,
#6997,#6998,#6999,#7000));
#7583=AXIS2_PLACEMENT_3D('',#13877,#8820,#8821);
#7584=AXIS2_PLACEMENT_3D('',#13878,#8822,#8823);
#7585=AXIS2_PLACEMENT_3D('',#13880,#8824,#8825);
#7586=AXIS2_PLACEMENT_3D('',#13883,#8827,#8828);
#7587=AXIS2_PLACEMENT_3D('',#13884,#8829,#8830);
#7588=AXIS2_PLACEMENT_3D('',#13886,#8831,#8832);
#7589=AXIS2_PLACEMENT_3D('',#13889,#8834,#8835);
#7590=AXIS2_PLACEMENT_3D('',#13890,#8836,#8837);
#7591=AXIS2_PLACEMENT_3D('',#13892,#8838,#8839);
#7592=AXIS2_PLACEMENT_3D('',#13894,#8840,#8841);
#7593=AXIS2_PLACEMENT_3D('',#13895,#8842,#8843);
#7594=AXIS2_PLACEMENT_3D('',#13897,#8844,#8845);
#7595=AXIS2_PLACEMENT_3D('',#13899,#8847,#8848);
#7596=AXIS2_PLACEMENT_3D('',#13900,#8849,#8850);
#7597=AXIS2_PLACEMENT_3D('',#13902,#8851,#8852);
#7598=AXIS2_PLACEMENT_3D('',#13904,#8853,#8854);
#7599=AXIS2_PLACEMENT_3D('',#13905,#8855,#8856);
#7600=AXIS2_PLACEMENT_3D('',#13907,#8857,#8858);
#7601=AXIS2_PLACEMENT_3D('',#13909,#8860,#8861);
#7602=AXIS2_PLACEMENT_3D('',#13910,#8862,#8863);
#7603=AXIS2_PLACEMENT_3D('',#13912,#8864,#8865);
#7604=AXIS2_PLACEMENT_3D('',#13914,#8866,#8867);
#7605=AXIS2_PLACEMENT_3D('',#13915,#8868,#8869);
#7606=AXIS2_PLACEMENT_3D('',#13917,#8870,#8871);
#7607=AXIS2_PLACEMENT_3D('',#13919,#8873,#8874);
#7608=AXIS2_PLACEMENT_3D('',#13920,#8875,#8876);
#7609=AXIS2_PLACEMENT_3D('',#13922,#8877,#8878);
#7610=AXIS2_PLACEMENT_3D('',#13924,#8879,#8880);
#7611=AXIS2_PLACEMENT_3D('',#13925,#8881,#8882);
#7612=AXIS2_PLACEMENT_3D('',#13927,#8883,#8884);
#7613=AXIS2_PLACEMENT_3D('',#13929,#8886,#8887);
#7614=AXIS2_PLACEMENT_3D('',#13930,#8888,#8889);
#7615=AXIS2_PLACEMENT_3D('',#13933,#8891,#8892);
#7616=AXIS2_PLACEMENT_3D('',#13934,#8893,#8894);
#7617=AXIS2_PLACEMENT_3D('',#13937,#8896,#8897);
#7618=AXIS2_PLACEMENT_3D('',#13938,#8898,#8899);
#7619=AXIS2_PLACEMENT_3D('',#13941,#8901,#8902);
#7620=AXIS2_PLACEMENT_3D('',#13942,#8903,#8904);
#7621=AXIS2_PLACEMENT_3D('',#13945,#8906,#8907);
#7622=AXIS2_PLACEMENT_3D('',#13973,#8908,#8909);
#7623=AXIS2_PLACEMENT_3D('',#13981,#8910,#8911);
#7624=AXIS2_PLACEMENT_3D('',#13987,#8912,#8913);
#7625=AXIS2_PLACEMENT_3D('',#13990,#8914,#8915);
#7626=AXIS2_PLACEMENT_3D('',#14020,#8918,#8919);
#7627=AXIS2_PLACEMENT_3D('',#14058,#8920,#8921);
#7628=AXIS2_PLACEMENT_3D('',#14096,#8922,#8923);
#7629=AXIS2_PLACEMENT_3D('',#14107,#8924,#8925);
#7630=AXIS2_PLACEMENT_3D('',#14110,#8926,#8927);
#7631=AXIS2_PLACEMENT_3D('',#14140,#8930,#8931);
#7632=AXIS2_PLACEMENT_3D('',#14186,#8932,#8933);
#7633=AXIS2_PLACEMENT_3D('',#14339,#8935,#8936);
#7634=AXIS2_PLACEMENT_3D('',#14340,#8937,#8938);
#7635=AXIS2_PLACEMENT_3D('',#14463,#8940,#8941);
#8820=DIRECTION('axis',(0.,0.,1.));
#8821=DIRECTION('refdir',(1.,0.,0.));
#8822=DIRECTION('center_axis',(0.,0.,-1.));
#8823=DIRECTION('ref_axis',(1.,0.,0.));
#8824=DIRECTION('center_axis',(-6.04309184969008E-32,-6.38489691472444E-32,
-1.));
#8825=DIRECTION('ref_axis',(1.,0.,0.));
#8826=DIRECTION('',(0.,0.,-1.));
#8827=DIRECTION('center_axis',(1.44549646912992E-31,1.50240180416177E-18,
1.));
#8828=DIRECTION('ref_axis',(1.,0.,0.));
#8829=DIRECTION('center_axis',(0.,0.,-1.));
#8830=DIRECTION('ref_axis',(1.,0.,0.));
#8831=DIRECTION('center_axis',(-6.04309184969008E-32,-6.38489691472444E-32,
-1.));
#8832=DIRECTION('ref_axis',(1.,0.,0.));
#8833=DIRECTION('',(0.,0.,-1.));
#8834=DIRECTION('center_axis',(1.44549646912992E-31,1.50240180416177E-18,
1.));
#8835=DIRECTION('ref_axis',(1.,0.,0.));
#8836=DIRECTION('center_axis',(0.,0.,1.));
#8837=DIRECTION('ref_axis',(1.,0.,0.));
#8838=DIRECTION('center_axis',(0.,0.,1.));
#8839=DIRECTION('ref_axis',(1.,0.,0.));
#8840=DIRECTION('center_axis',(0.,0.,-1.));
#8841=DIRECTION('ref_axis',(1.,0.,0.));
#8842=DIRECTION('center_axis',(0.,0.,-1.));
#8843=DIRECTION('ref_axis',(1.,0.,0.));
#8844=DIRECTION('center_axis',(0.,0.,-1.));
#8845=DIRECTION('ref_axis',(1.,0.,0.));
#8846=DIRECTION('',(0.,0.,1.));
#8847=DIRECTION('center_axis',(0.,0.,1.));
#8848=DIRECTION('ref_axis',(1.,0.,0.));
#8849=DIRECTION('center_axis',(0.,0.,1.));
#8850=DIRECTION('ref_axis',(1.,0.,0.));
#8851=DIRECTION('center_axis',(0.,0.,1.));
#8852=DIRECTION('ref_axis',(1.,0.,0.));
#8853=DIRECTION('center_axis',(0.,0.,-1.));
#8854=DIRECTION('ref_axis',(1.,0.,0.));
#8855=DIRECTION('center_axis',(0.,0.,-1.));
#8856=DIRECTION('ref_axis',(1.,0.,0.));
#8857=DIRECTION('center_axis',(0.,0.,-1.));
#8858=DIRECTION('ref_axis',(1.,0.,0.));
#8859=DIRECTION('',(0.,0.,1.));
#8860=DIRECTION('center_axis',(0.,0.,1.));
#8861=DIRECTION('ref_axis',(1.,0.,0.));
#8862=DIRECTION('center_axis',(0.,0.,1.));
#8863=DIRECTION('ref_axis',(1.,0.,0.));
#8864=DIRECTION('center_axis',(0.,0.,1.));
#8865=DIRECTION('ref_axis',(1.,0.,0.));
#8866=DIRECTION('center_axis',(0.,0.,-1.));
#8867=DIRECTION('ref_axis',(1.,0.,0.));
#8868=DIRECTION('center_axis',(0.,0.,-1.));
#8869=DIRECTION('ref_axis',(1.,0.,0.));
#8870=DIRECTION('center_axis',(0.,0.,-1.));
#8871=DIRECTION('ref_axis',(1.,0.,0.));
#8872=DIRECTION('',(0.,0.,1.));
#8873=DIRECTION('center_axis',(0.,0.,1.));
#8874=DIRECTION('ref_axis',(1.,0.,0.));
#8875=DIRECTION('center_axis',(0.,0.,1.));
#8876=DIRECTION('ref_axis',(1.,0.,0.));
#8877=DIRECTION('center_axis',(0.,0.,1.));
#8878=DIRECTION('ref_axis',(1.,0.,0.));
#8879=DIRECTION('center_axis',(0.,0.,-1.));
#8880=DIRECTION('ref_axis',(1.,0.,0.));
#8881=DIRECTION('center_axis',(0.,0.,-1.));
#8882=DIRECTION('ref_axis',(1.,0.,0.));
#8883=DIRECTION('center_axis',(0.,0.,-1.));
#8884=DIRECTION('ref_axis',(1.,0.,0.));
#8885=DIRECTION('',(0.,0.,1.));
#8886=DIRECTION('center_axis',(0.,0.,1.));
#8887=DIRECTION('ref_axis',(1.,0.,0.));
#8888=DIRECTION('center_axis',(0.,0.,-1.));
#8889=DIRECTION('ref_axis',(1.,0.,0.));
#8890=DIRECTION('',(0.,0.,1.));
#8891=DIRECTION('center_axis',(1.44549646912992E-31,1.50240180416177E-18,
1.));
#8892=DIRECTION('ref_axis',(1.,0.,0.));
#8893=DIRECTION('center_axis',(0.,0.,-1.));
#8894=DIRECTION('ref_axis',(1.,0.,0.));
#8895=DIRECTION('',(0.,0.,1.));
#8896=DIRECTION('center_axis',(1.44549646912992E-31,1.50240180416177E-18,
1.));
#8897=DIRECTION('ref_axis',(1.,0.,0.));
#8898=DIRECTION('center_axis',(0.,0.,-1.));
#8899=DIRECTION('ref_axis',(1.,0.,0.));
#8900=DIRECTION('',(0.,0.,1.));
#8901=DIRECTION('center_axis',(1.44549646912992E-31,1.50240180416177E-18,
1.));
#8902=DIRECTION('ref_axis',(1.,0.,0.));
#8903=DIRECTION('center_axis',(0.,0.,-1.));
#8904=DIRECTION('ref_axis',(1.,0.,0.));
#8905=DIRECTION('',(0.,0.,1.));
#8906=DIRECTION('center_axis',(1.44549646912992E-31,1.50240180416177E-18,
1.));
#8907=DIRECTION('ref_axis',(1.,0.,0.));
#8908=DIRECTION('center_axis',(0.,1.,0.));
#8909=DIRECTION('ref_axis',(0.,0.,1.));
#8910=DIRECTION('center_axis',(0.993165917563083,0.116711011438853,0.));
#8911=DIRECTION('ref_axis',(-0.116587207627638,0.992112394641407,0.0460480120795941));
#8912=DIRECTION('center_axis',(-3.34618268251883E-33,-1.,6.38489691472444E-32));
#8913=DIRECTION('ref_axis',(0.688354575693762,0.,0.72537437101228));
#8914=DIRECTION('center_axis',(0.,1.,0.));
#8915=DIRECTION('ref_axis',(0.,0.,1.));
#8916=DIRECTION('',(3.34618268251883E-33,1.,-6.38489691472444E-32));
#8917=DIRECTION('',(-3.34618268251883E-33,-1.,6.38489691472444E-32));
#8918=DIRECTION('center_axis',(0.993165917563077,-0.116711011438899,0.));
#8919=DIRECTION('ref_axis',(0.,0.,1.));
#8920=DIRECTION('center_axis',(0.999711469489423,-0.0240203615980049,0.));
#8921=DIRECTION('ref_axis',(0.,0.,1.));
#8922=DIRECTION('center_axis',(-3.69655756055634E-12,-1.,2.05200165779092E-26));
#8923=DIRECTION('ref_axis',(5.55111512312576E-15,0.,1.));
#8924=DIRECTION('center_axis',(-3.3461826825185E-33,1.,-6.38489691472444E-32));
#8925=DIRECTION('ref_axis',(-0.688354575693751,0.,0.72537437101229));
#8926=DIRECTION('center_axis',(0.,-1.,0.));
#8927=DIRECTION('ref_axis',(0.,0.,1.));
#8928=DIRECTION('',(3.3461826825185E-33,-1.,6.38489691472444E-32));
#8929=DIRECTION('',(-3.3461826825185E-33,1.,-6.38489691472444E-32));
#8930=DIRECTION('center_axis',(-0.999711469481833,-0.0240203619138888,2.77475672850144E-15));
#8931=DIRECTION('ref_axis',(2.77555756156288E-15,0.,1.));
#8932=DIRECTION('center_axis',(0.998629534754574,0.,-0.0523359562429439));
#8933=DIRECTION('ref_axis',(-0.0523359562429439,0.,-0.998629534754574));
#8934=DIRECTION('',(0.,1.,0.));
#8935=DIRECTION('center_axis',(6.04309184969008E-32,6.38489691472444E-32,
1.));
#8936=DIRECTION('ref_axis',(1.,0.,-6.04309184969008E-32));
#8937=DIRECTION('center_axis',(-0.998629534754574,0.,-0.0523359562429491));
#8938=DIRECTION('ref_axis',(-0.0523359562429491,0.,0.998629534754574));
#8939=DIRECTION('',(0.,-1.,0.));
#8940=DIRECTION('center_axis',(1.44549646912992E-31,1.50240180416177E-18,
1.));
#8941=DIRECTION('ref_axis',(1.,0.,-1.44549646912992E-31));
#13877=CARTESIAN_POINT('',(0.,0.,0.));
#13878=CARTESIAN_POINT('Origin',(2.,0.,1.));
#13879=CARTESIAN_POINT('',(1.65,4.28626379701574E-17,1.1));
#13880=CARTESIAN_POINT('Origin',(2.,0.,1.1));
#13881=CARTESIAN_POINT('',(1.65,4.28626379701574E-17,0.9));
#13882=CARTESIAN_POINT('',(1.65,4.28626379701574E-17,1.));
#13883=CARTESIAN_POINT('Origin',(2.,0.,0.9));
#13884=CARTESIAN_POINT('Origin',(11.2,0.,1.));
#13885=CARTESIAN_POINT('',(10.85,4.28626379701574E-17,1.1));
#13886=CARTESIAN_POINT('Origin',(11.2,0.,1.1));
#13887=CARTESIAN_POINT('',(10.85,4.28626379701574E-17,0.9));
#13888=CARTESIAN_POINT('',(10.85,4.28626379701574E-17,1.));
#13889=CARTESIAN_POINT('Origin',(11.2,0.,0.9));
#13890=CARTESIAN_POINT('Origin',(9.9,1.,0.7));
#13891=CARTESIAN_POINT('',(9.65,1.,0.7));
#13892=CARTESIAN_POINT('Origin',(9.9,1.,0.7));
#13893=CARTESIAN_POINT('',(9.75,1.,0.7));
#13894=CARTESIAN_POINT('Origin',(9.9,1.,0.7));
#13895=CARTESIAN_POINT('Origin',(9.9,1.,0.7));
#13896=CARTESIAN_POINT('',(9.65,1.,0.6));
#13897=CARTESIAN_POINT('Origin',(9.9,1.,0.6));
#13898=CARTESIAN_POINT('',(9.65,1.,0.7));
#13899=CARTESIAN_POINT('Origin',(9.9,1.,0.6));
#13900=CARTESIAN_POINT('Origin',(3.3,-1.,0.7));
#13901=CARTESIAN_POINT('',(3.05,-1.,0.7));
#13902=CARTESIAN_POINT('Origin',(3.3,-1.,0.7));
#13903=CARTESIAN_POINT('',(3.15,-1.,0.7));
#13904=CARTESIAN_POINT('Origin',(3.3,-1.,0.7));
#13905=CARTESIAN_POINT('Origin',(3.3,-1.,0.7));
#13906=CARTESIAN_POINT('',(3.05,-1.,0.6));
#13907=CARTESIAN_POINT('Origin',(3.3,-1.,0.6));
#13908=CARTESIAN_POINT('',(3.05,-1.,0.7));
#13909=CARTESIAN_POINT('Origin',(3.3,-1.,0.6));
#13910=CARTESIAN_POINT('Origin',(3.3,1.,0.7));
#13911=CARTESIAN_POINT('',(3.05,1.,0.7));
#13912=CARTESIAN_POINT('Origin',(3.3,1.,0.7));
#13913=CARTESIAN_POINT('',(3.15,1.,0.7));
#13914=CARTESIAN_POINT('Origin',(3.3,1.,0.7));
#13915=CARTESIAN_POINT('Origin',(3.3,1.,0.7));
#13916=CARTESIAN_POINT('',(3.05,1.,0.6));
#13917=CARTESIAN_POINT('Origin',(3.3,1.,0.6));
#13918=CARTESIAN_POINT('',(3.05,1.,0.7));
#13919=CARTESIAN_POINT('Origin',(3.3,1.,0.6));
#13920=CARTESIAN_POINT('Origin',(9.9,-1.,0.7));
#13921=CARTESIAN_POINT('',(9.65,-1.,0.7));
#13922=CARTESIAN_POINT('Origin',(9.9,-1.,0.7));
#13923=CARTESIAN_POINT('',(9.75,-1.,0.7));
#13924=CARTESIAN_POINT('Origin',(9.9,-1.,0.7));
#13925=CARTESIAN_POINT('Origin',(9.9,-1.,0.7));
#13926=CARTESIAN_POINT('',(9.65,-1.,0.6));
#13927=CARTESIAN_POINT('Origin',(9.9,-1.,0.6));
#13928=CARTESIAN_POINT('',(9.65,-1.,0.7));
#13929=CARTESIAN_POINT('Origin',(9.9,-1.,0.6));
#13930=CARTESIAN_POINT('Origin',(9.9,1.,0.9));
#13931=CARTESIAN_POINT('',(9.75,1.,0.9));
#13932=CARTESIAN_POINT('',(9.75,1.,0.9));
#13933=CARTESIAN_POINT('Origin',(9.9,1.,0.9));
#13934=CARTESIAN_POINT('Origin',(3.3,-1.,0.9));
#13935=CARTESIAN_POINT('',(3.15,-1.,0.9));
#13936=CARTESIAN_POINT('',(3.15,-1.,0.9));
#13937=CARTESIAN_POINT('Origin',(3.3,-1.,0.9));
#13938=CARTESIAN_POINT('Origin',(3.3,1.,0.9));
#13939=CARTESIAN_POINT('',(3.15,1.,0.9));
#13940=CARTESIAN_POINT('',(3.15,1.,0.9));
#13941=CARTESIAN_POINT('Origin',(3.3,1.,0.9));
#13942=CARTESIAN_POINT('Origin',(9.9,-1.,0.9));
#13943=CARTESIAN_POINT('',(9.75,-1.,0.9));
#13944=CARTESIAN_POINT('',(9.75,-1.,0.9));
#13945=CARTESIAN_POINT('Origin',(9.9,-1.,0.9));
#13946=CARTESIAN_POINT('Ctrl Pts',(12.6883460378814,1.74710477827991,1.1));
#13947=CARTESIAN_POINT('Ctrl Pts',(12.7050904406715,1.74907248191433,1.1));
#13948=CARTESIAN_POINT('Ctrl Pts',(12.7459721545883,1.73893278412019,1.1));
#13949=CARTESIAN_POINT('Ctrl Pts',(12.7664342774515,1.70015954799943,1.1));
#13950=CARTESIAN_POINT('Ctrl Pts',(12.7664342774515,1.67768005087614,1.1));
#13951=CARTESIAN_POINT('Ctrl Pts',(12.6856343728622,1.77018000694724,1.1));
#13952=CARTESIAN_POINT('Ctrl Pts',(12.70797027111,1.77258660535003,1.09999193474305));
#13953=CARTESIAN_POINT('Ctrl Pts',(12.7620607807224,1.75878051965913,1.09998076816122));
#13954=CARTESIAN_POINT('Ctrl Pts',(12.789311301819,1.70760782583852,1.09999039212455));
#13955=CARTESIAN_POINT('Ctrl Pts',(12.7895723566779,1.67768005087614,1.1));
#13956=CARTESIAN_POINT('Ctrl Pts',(12.6809355967604,1.81016478834023,1.08112516654061));
#13957=CARTESIAN_POINT('Ctrl Pts',(12.7128933108791,1.81335099699619,1.08149246505882));
#13958=CARTESIAN_POINT('Ctrl Pts',(12.7898658458254,1.7931743676233,1.08208124913004));
#13959=CARTESIAN_POINT('Ctrl Pts',(12.8289908274994,1.72043204305838,1.08173005449524));
#13960=CARTESIAN_POINT('Ctrl Pts',(12.829672543413,1.67768005087614,1.08128963884528));
#13961=CARTESIAN_POINT('Ctrl Pts',(12.6791127113589,1.82567684354491,1.04109086533338));
#13962=CARTESIAN_POINT('Ctrl Pts',(12.7147851087716,1.82957775596959,1.04203732134162));
#13963=CARTESIAN_POINT('Ctrl Pts',(12.8014031907485,1.80754024306994,1.04357783697133));
#13964=CARTESIAN_POINT('Ctrl Pts',(12.8450621014111,1.72550665092358,1.04265503156396));
#13965=CARTESIAN_POINT('Ctrl Pts',(12.8454164251054,1.67768005087614,1.0415166534692));
#13966=CARTESIAN_POINT('Ctrl Pts',(12.6790190612712,1.82647376985122,1.02368384096639));
#13967=CARTESIAN_POINT('Ctrl Pts',(12.7148414907177,1.83063166001164,1.02479882190871));
#13968=CARTESIAN_POINT('Ctrl Pts',(12.8023492944496,1.80880756543048,1.02662811038865));
#13969=CARTESIAN_POINT('Ctrl Pts',(12.8462542441509,1.7257797841646,1.02553011374107));
#13970=CARTESIAN_POINT('Ctrl Pts',(12.8463246402318,1.67768005087614,1.02418687649944));
#13971=CARTESIAN_POINT('',(12.7664342774515,1.67768005087614,1.1));
#13972=CARTESIAN_POINT('',(12.8463246402318,1.67768005087614,1.02418687649944));
#13973=CARTESIAN_POINT('Origin',(12.7664342774515,1.67768005087614,1.02));
#13974=CARTESIAN_POINT('',(12.6790190612712,1.82647376985123,1.02368384096637));
#13975=CARTESIAN_POINT('Ctrl Pts',(12.8463246402318,1.67768005087614,1.02418687649944));
#13976=CARTESIAN_POINT('Ctrl Pts',(12.8462542441509,1.7257797841646,1.02553011374107));
#13977=CARTESIAN_POINT('Ctrl Pts',(12.8023492944496,1.80880756543048,1.02662811038865));
#13978=CARTESIAN_POINT('Ctrl Pts',(12.7148414907177,1.83063166001164,1.02479882190871));
#13979=CARTESIAN_POINT('Ctrl Pts',(12.6790190612712,1.82647376985122,1.02368384096639));
#13980=CARTESIAN_POINT('',(12.6883460378814,1.74710477827991,1.1));
#13981=CARTESIAN_POINT('Origin',(12.6883460378814,1.74710477827991,1.02));
#13982=CARTESIAN_POINT('Ctrl Pts',(12.6883460378814,1.74710477827991,1.1));
#13983=CARTESIAN_POINT('Ctrl Pts',(12.7050904406715,1.74907248191433,1.1));
#13984=CARTESIAN_POINT('Ctrl Pts',(12.7459721545883,1.73893278412019,1.1));
#13985=CARTESIAN_POINT('Ctrl Pts',(12.7664342774515,1.70015954799943,1.1));
#13986=CARTESIAN_POINT('Ctrl Pts',(12.7664342774515,1.67768005087614,1.1));
#13987=CARTESIAN_POINT('Origin',(12.7664342774515,0.926416499322631,1.02));
#13988=CARTESIAN_POINT('',(12.7664342774515,-1.67768005087614,1.1));
#13989=CARTESIAN_POINT('',(12.8463246402318,-1.67768005087614,1.02418687649944));
#13990=CARTESIAN_POINT('Origin',(12.7664342774515,-1.67768005087614,1.02));
#13991=CARTESIAN_POINT('',(12.8463246402318,0.926416499322631,1.02418687649944));
#13992=CARTESIAN_POINT('',(12.7664342774515,0.926416499322631,1.1));
#13993=CARTESIAN_POINT('Ctrl Pts',(12.7664342774515,-1.67768005087614,1.1));
#13994=CARTESIAN_POINT('Ctrl Pts',(12.7664342774515,-1.69453967371875,1.1));
#13995=CARTESIAN_POINT('Ctrl Pts',(12.7515713182712,-1.73395715258217,1.1));
#13996=CARTESIAN_POINT('Ctrl Pts',(12.7106719082684,-1.74972838312583,1.1));
#13997=CARTESIAN_POINT('Ctrl Pts',(12.6883460378814,-1.74710477827991,1.1));
#13998=CARTESIAN_POINT('Ctrl Pts',(12.7895723566779,-1.67768005087614,1.1));
#13999=CARTESIAN_POINT('Ctrl Pts',(12.7893765655337,-1.70012588209812,1.09999279409341));
#14000=CARTESIAN_POINT('Ctrl Pts',(12.7694119126837,-1.75223468493452,1.09998162170574));
#14001=CARTESIAN_POINT('Ctrl Pts',(12.7154155705261,-1.77338880481765,1.09998924632407));
#14002=CARTESIAN_POINT('Ctrl Pts',(12.6856343728622,-1.77018000694724,1.1));
#14003=CARTESIAN_POINT('Ctrl Pts',(12.829672543413,-1.67768005087614,1.08128963884528));
#14004=CARTESIAN_POINT('Ctrl Pts',(12.8291612564778,-1.70974404501309,1.08161995058275));
#14005=CARTESIAN_POINT('Ctrl Pts',(12.800330508486,-1.78383870138124,1.08209231231141));
#14006=CARTESIAN_POINT('Ctrl Pts',(12.7235458822523,-1.81441306654821,1.08161489789823));
#14007=CARTESIAN_POINT('Ctrl Pts',(12.6809355967604,-1.81016478834023,1.08112516654061));
#14008=CARTESIAN_POINT('Ctrl Pts',(12.8454164251054,-1.67768005087614,1.0415166534692));
#14009=CARTESIAN_POINT('Ctrl Pts',(12.8451506823347,-1.71355000091203,1.04237043704028));
#14010=CARTESIAN_POINT('Ctrl Pts',(12.8132193893781,-1.79702133948082,1.04360777159741));
#14011=CARTESIAN_POINT('Ctrl Pts',(12.7266759079096,-1.8308780601112,1.04235280667771));
#14012=CARTESIAN_POINT('Ctrl Pts',(12.6791127113589,-1.82567684354491,1.04109086533338));
#14013=CARTESIAN_POINT('Ctrl Pts',(12.8463246402318,-1.67768005087614,1.02418687649944));
#14014=CARTESIAN_POINT('Ctrl Pts',(12.8462718431712,-1.71375485084279,1.02519430443067));
#14015=CARTESIAN_POINT('Ctrl Pts',(12.8143456047297,-1.79814359426379,1.02666431898144));
#14016=CARTESIAN_POINT('Ctrl Pts',(12.7267823005336,-1.83201762339849,1.02517048222283));
#14017=CARTESIAN_POINT('Ctrl Pts',(12.6790190612712,-1.82647376985122,1.02368384096639));
#14018=CARTESIAN_POINT('',(12.6883460378814,-1.74710477827991,1.1));
#14019=CARTESIAN_POINT('',(12.6790190612712,-1.82647376985122,1.02368384096639));
#14020=CARTESIAN_POINT('Origin',(12.6883460378814,-1.74710477827991,1.02));
#14021=CARTESIAN_POINT('Ctrl Pts',(12.6790190612712,-1.82647376985122,1.02368384096639));
#14022=CARTESIAN_POINT('Ctrl Pts',(12.7267823005336,-1.83201762339849,1.02517048222283));
#14023=CARTESIAN_POINT('Ctrl Pts',(12.8143456047297,-1.79814359426379,1.02666431898144));
#14024=CARTESIAN_POINT('Ctrl Pts',(12.8462718431712,-1.71375485084279,1.02519430443067));
#14025=CARTESIAN_POINT('Ctrl Pts',(12.8463246402318,-1.67768005087614,1.02418687649944));
#14026=CARTESIAN_POINT('Ctrl Pts',(12.7664342774515,-1.67768005087614,1.1));
#14027=CARTESIAN_POINT('Ctrl Pts',(12.7664342774515,-1.69453967371875,1.1));
#14028=CARTESIAN_POINT('Ctrl Pts',(12.7515713182712,-1.73395715258217,1.1));
#14029=CARTESIAN_POINT('Ctrl Pts',(12.7106719082684,-1.74972838312583,1.1));
#14030=CARTESIAN_POINT('Ctrl Pts',(12.6883460378814,-1.74710477827991,1.1));
#14031=CARTESIAN_POINT('Ctrl Pts',(12.6883460378814,-1.74710477827991,1.1));
#14032=CARTESIAN_POINT('Ctrl Pts',(10.9559705848985,-1.54352621428166,1.1));
#14033=CARTESIAN_POINT('Ctrl Pts',(6.89625808461774,-1.22619725057464,1.1));
#14034=CARTESIAN_POINT('Ctrl Pts',(2.82684345252479,-1.12583341467021,1.1));
#14035=CARTESIAN_POINT('Ctrl Pts',(0.501786340825443,-1.06996858265586,
1.1));
#14036=CARTESIAN_POINT('Ctrl Pts',(12.6856343728622,-1.77018000694724,1.1));
#14037=CARTESIAN_POINT('Ctrl Pts',(10.953864459251,-1.56662322149928,1.09999817462394));
#14038=CARTESIAN_POINT('Ctrl Pts',(6.89527069668598,-1.24931220526659,1.1000008953949));
#14039=CARTESIAN_POINT('Ctrl Pts',(2.8262782431937,-1.14895306774358,1.10000025453557));
#14040=CARTESIAN_POINT('Ctrl Pts',(0.501230998995504,-1.09308153985212,
1.1));
#14041=CARTESIAN_POINT('Ctrl Pts',(12.6809355941985,-1.8101648101409,1.08112518582372));
#14042=CARTESIAN_POINT('Ctrl Pts',(10.9502073547204,-1.60665097561358,1.08120831496985));
#14043=CARTESIAN_POINT('Ctrl Pts',(6.89356335983392,-1.28937229578717,1.08131090328882));
#14044=CARTESIAN_POINT('Ctrl Pts',(2.82529878789426,-1.18902174359502,1.08130951558098));
#14045=CARTESIAN_POINT('Ctrl Pts',(0.500268515819014,-1.13313944880305,
1.0813211979534));
#14046=CARTESIAN_POINT('Ctrl Pts',(12.6791127113589,-1.82567684354491,1.04109086533338));
#14047=CARTESIAN_POINT('Ctrl Pts',(10.9487809439014,-1.62227255850559,1.04130507278566));
#14048=CARTESIAN_POINT('Ctrl Pts',(6.89288912441654,-1.30512519378816,1.04157208078929));
#14049=CARTESIAN_POINT('Ctrl Pts',(2.82491362604336,-1.2047760518259,1.04156824165415));
#14050=CARTESIAN_POINT('Ctrl Pts',(0.499889770467655,-1.14890257814483,
1.04159845594383));
#14051=CARTESIAN_POINT('Ctrl Pts',(12.6790190612712,-1.82647376985122,1.02368384096639));
#14052=CARTESIAN_POINT('Ctrl Pts',(10.9487001718726,-1.62312516854374,1.02393618996614));
#14053=CARTESIAN_POINT('Ctrl Pts',(6.89285005483575,-1.30604661809728,1.02425267661394));
#14054=CARTESIAN_POINT('Ctrl Pts',(2.82489114035621,-1.20569670918473,1.0242479474763));
#14055=CARTESIAN_POINT('Ctrl Pts',(0.499867468581681,-1.14983076778971,
1.024283610038));
#14056=CARTESIAN_POINT('',(0.501786340825443,-1.06996858265586,1.1));
#14057=CARTESIAN_POINT('',(0.499867468607324,-1.1498307677904,1.02428361003669));
#14058=CARTESIAN_POINT('Origin',(0.501786340825443,-1.06996858265586,1.02));
#14059=CARTESIAN_POINT('Ctrl Pts',(0.499867468581681,-1.14983076778971,
1.024283610038));
#14060=CARTESIAN_POINT('Ctrl Pts',(2.82489114035621,-1.20569670918473,1.0242479474763));
#14061=CARTESIAN_POINT('Ctrl Pts',(6.89285005483575,-1.30604661809728,1.02425267661394));
#14062=CARTESIAN_POINT('Ctrl Pts',(10.9487001718726,-1.62312516854374,1.02393618996614));
#14063=CARTESIAN_POINT('Ctrl Pts',(12.6790190612712,-1.82647376985122,1.02368384096639));
#14064=CARTESIAN_POINT('Ctrl Pts',(12.6883460378814,-1.74710477827991,1.1));
#14065=CARTESIAN_POINT('Ctrl Pts',(10.9559705848985,-1.54352621428166,1.1));
#14066=CARTESIAN_POINT('Ctrl Pts',(6.89625808461774,-1.22619725057464,1.1));
#14067=CARTESIAN_POINT('Ctrl Pts',(2.82684345252479,-1.12583341467021,1.1));
#14068=CARTESIAN_POINT('Ctrl Pts',(0.501786340825443,-1.06996858265586,
1.1));
#14069=CARTESIAN_POINT('Ctrl Pts',(0.501786340845132,-1.06996858265633,
1.1));
#14070=CARTESIAN_POINT('Ctrl Pts',(0.486343670353271,-1.06959753705714,
1.1));
#14071=CARTESIAN_POINT('Ctrl Pts',(0.450546621606563,-1.05636265633066,
1.1));
#14072=CARTESIAN_POINT('Ctrl Pts',(0.4335657225485,-1.02068090721437,1.1));
#14073=CARTESIAN_POINT('Ctrl Pts',(0.433565722548536,-1.00008473726807,
1.1));
#14074=CARTESIAN_POINT('Ctrl Pts',(0.501230999004731,-1.09308153985199,
1.1));
#14075=CARTESIAN_POINT('Ctrl Pts',(0.480678852604012,-1.0924131923446,1.09999359215549));
#14076=CARTESIAN_POINT('Ctrl Pts',(0.433334506735602,-1.0746197149398,1.09998454864803));
#14077=CARTESIAN_POINT('Ctrl Pts',(0.410665947227687,-1.02750530853182,
1.09999122945172));
#14078=CARTESIAN_POINT('Ctrl Pts',(0.410427643322096,-1.00008473726803,
1.1));
#14079=CARTESIAN_POINT('Ctrl Pts',(0.500268097562941,-1.13315685597024,
1.08133662520967));
#14080=CARTESIAN_POINT('Ctrl Pts',(0.470917694462572,-1.13199579109467,
1.08163072487897));
#14081=CARTESIAN_POINT('Ctrl Pts',(0.403559863183325,-1.10627672518437,
1.08206304806334));
#14082=CARTESIAN_POINT('Ctrl Pts',(0.370932263602498,-1.0392553542177,1.08170715357768));
#14083=CARTESIAN_POINT('Ctrl Pts',(0.370309959289207,-1.00008473726796,
1.08130512018932));
#14084=CARTESIAN_POINT('Ctrl Pts',(0.4998897704516,-1.14890257814396,1.04159845594539));
#14085=CARTESIAN_POINT('Ctrl Pts',(0.467042111092653,-1.1478756708603,1.04235909019736));
#14086=CARTESIAN_POINT('Ctrl Pts',(0.391210771603448,-1.11942230347982,
1.04349095641912));
#14087=CARTESIAN_POINT('Ctrl Pts',(0.354907019248534,-1.04390490695311,
1.04255582181557));
#14088=CARTESIAN_POINT('Ctrl Pts',(0.354583574894623,-1.00008473726793,
1.04151665346919));
#14089=CARTESIAN_POINT('Ctrl Pts',(0.499867468565196,-1.14983076778922,
1.02428361003984));
#14090=CARTESIAN_POINT('Ctrl Pts',(0.466823083113769,-1.14898864521809,
1.02518140264794));
#14091=CARTESIAN_POINT('Ctrl Pts',(0.390185579422885,-1.12055776822857,
1.0265258196442));
#14092=CARTESIAN_POINT('Ctrl Pts',(0.353739620824501,-1.04415516223227,
1.0254130505005));
#14093=CARTESIAN_POINT('Ctrl Pts',(0.353675359768169,-1.00008473726793,
1.02418687649943));
#14094=CARTESIAN_POINT('',(0.433565722548536,-1.00008473726807,1.1));
#14095=CARTESIAN_POINT('',(0.353675359768456,-1.00008473726778,1.0241868765049));
#14096=CARTESIAN_POINT('Origin',(0.433565722548536,-1.00008473726807,1.02));
#14097=CARTESIAN_POINT('Ctrl Pts',(0.353675359768169,-1.00008473726793,
1.02418687649943));
#14098=CARTESIAN_POINT('Ctrl Pts',(0.353739620824501,-1.04415516223227,
1.0254130505005));
#14099=CARTESIAN_POINT('Ctrl Pts',(0.390185579422885,-1.12055776822857,
1.0265258196442));
#14100=CARTESIAN_POINT('Ctrl Pts',(0.466823083113769,-1.14898864521809,
1.02518140264794));
#14101=CARTESIAN_POINT('Ctrl Pts',(0.499867468565196,-1.14983076778922,
1.02428361003984));
#14102=CARTESIAN_POINT('Ctrl Pts',(0.501786340845132,-1.06996858265633,
1.1));
#14103=CARTESIAN_POINT('Ctrl Pts',(0.486343670353271,-1.06959753705714,
1.1));
#14104=CARTESIAN_POINT('Ctrl Pts',(0.450546621606563,-1.05636265633066,
1.1));
#14105=CARTESIAN_POINT('Ctrl Pts',(0.4335657225485,-1.02068090721437,1.1));
#14106=CARTESIAN_POINT('Ctrl Pts',(0.433565722548536,-1.00008473726807,
1.1));
#14107=CARTESIAN_POINT('Origin',(0.433565722548535,-0.576416499322632,1.02));
#14108=CARTESIAN_POINT('',(0.433565722548535,1.0000847372682,1.1));
#14109=CARTESIAN_POINT('',(0.35367535976817,1.0000847372682,1.02418687649944));
#14110=CARTESIAN_POINT('Origin',(0.433565722548535,1.0000847372682,1.02));
#14111=CARTESIAN_POINT('',(0.35367535976817,-0.576416499322632,1.02418687649944));
#14112=CARTESIAN_POINT('',(0.433565722548535,-0.576416499322632,1.1));
#14113=CARTESIAN_POINT('Ctrl Pts',(0.433565722548535,1.0000847372682,1.1));
#14114=CARTESIAN_POINT('Ctrl Pts',(0.433565722548535,1.01553186472631,1.1));
#14115=CARTESIAN_POINT('Ctrl Pts',(0.445933851022605,1.05163704585376,1.1));
#14116=CARTESIAN_POINT('Ctrl Pts',(0.481196113556474,1.06947385520094,1.1));
#14117=CARTESIAN_POINT('Ctrl Pts',(0.501786340877041,1.0699685826571,1.1));
#14118=CARTESIAN_POINT('Ctrl Pts',(0.410427643322096,1.0000847372682,1.1));
#14119=CARTESIAN_POINT('Ctrl Pts',(0.410606371251307,1.0206501657139,1.09999342208879));
#14120=CARTESIAN_POINT('Ctrl Pts',(0.427269489276852,1.06840883688971,1.09998438534344));
#14121=CARTESIAN_POINT('Ctrl Pts',(0.473828137181897,1.09219040985597,1.09999145620732));
#14122=CARTESIAN_POINT('Ctrl Pts',(0.501230999047159,1.09308153985336,1.1));
#14123=CARTESIAN_POINT('Ctrl Pts',(0.370309959289211,1.0000847372682,1.08130512018932));
#14124=CARTESIAN_POINT('Ctrl Pts',(0.370776687524182,1.02946269997745,1.08160664523056));
#14125=CARTESIAN_POINT('Ctrl Pts',(0.394906927696186,1.09741901043509,1.08206104999852));
#14126=CARTESIAN_POINT('Ctrl Pts',(0.461134226826275,1.13160876948958,1.08172875810162));
#14127=CARTESIAN_POINT('Ctrl Pts',(0.500268097623607,1.13315685597264,1.08133662520906));
#14128=CARTESIAN_POINT('Ctrl Pts',(0.354583574894625,1.0000847372682,1.0415166534692));
#14129=CARTESIAN_POINT('Ctrl Pts',(0.354826158160091,1.03294986452867,1.0422960297289));
#14130=CARTESIAN_POINT('Ctrl Pts',(0.381463759848658,1.10944036955345,1.04348552759116));
#14131=CARTESIAN_POINT('Ctrl Pts',(0.456092891378057,1.14753336845448,1.04261263494683));
#14132=CARTESIAN_POINT('Ctrl Pts',(0.499889770519448,1.14890257814608,1.04159845594382));
#14133=CARTESIAN_POINT('Ctrl Pts',(0.35367535976817,1.0000847372682,1.02418687649944));
#14134=CARTESIAN_POINT('Ctrl Pts',(0.353723555560473,1.03313755598801,1.02510650700014));
#14135=CARTESIAN_POINT('Ctrl Pts',(0.380300727059747,1.11043180383933,1.02651925632578));
#14136=CARTESIAN_POINT('Ctrl Pts',(0.455808288035698,1.1487079377163,1.02548066684923));
#14137=CARTESIAN_POINT('Ctrl Pts',(0.499867468633476,1.14983076779096,1.02428361003799));
#14138=CARTESIAN_POINT('',(0.501786340877041,1.0699685826571,1.1));
#14139=CARTESIAN_POINT('',(0.499867468633699,1.14983076779054,1.0242836100458));
#14140=CARTESIAN_POINT('Origin',(0.501786340877041,1.0699685826571,1.02));
#14141=CARTESIAN_POINT('Ctrl Pts',(0.499867468633476,1.14983076779096,1.02428361003799));
#14142=CARTESIAN_POINT('Ctrl Pts',(0.455808288035698,1.1487079377163,1.02548066684923));
#14143=CARTESIAN_POINT('Ctrl Pts',(0.380300727059747,1.11043180383933,1.02651925632578));
#14144=CARTESIAN_POINT('Ctrl Pts',(0.353723555560473,1.03313755598801,1.02510650700014));
#14145=CARTESIAN_POINT('Ctrl Pts',(0.35367535976817,1.0000847372682,1.02418687649944));
#14146=CARTESIAN_POINT('Ctrl Pts',(0.433565722548535,1.0000847372682,1.1));
#14147=CARTESIAN_POINT('Ctrl Pts',(0.433565722548535,1.01553186472631,1.1));
#14148=CARTESIAN_POINT('Ctrl Pts',(0.445933851022605,1.05163704585376,1.1));
#14149=CARTESIAN_POINT('Ctrl Pts',(0.481196113556474,1.06947385520094,1.1));
#14150=CARTESIAN_POINT('Ctrl Pts',(0.501786340877041,1.0699685826571,1.1));
#14151=CARTESIAN_POINT('Ctrl Pts',(0.501786340877248,1.0699685826571,1.1));
#14152=CARTESIAN_POINT('Ctrl Pts',(2.82684356715236,1.12583341742443,1.1));
#14153=CARTESIAN_POINT('Ctrl Pts',(6.89625445951469,1.22619710828032,1.1));
#14154=CARTESIAN_POINT('Ctrl Pts',(10.9559704995293,1.54352620424957,1.1));
#14155=CARTESIAN_POINT('Ctrl Pts',(12.6883460378814,1.74710477827991,1.1));
#14156=CARTESIAN_POINT('Ctrl Pts',(0.501230999047308,1.09308153985337,1.1));
#14157=CARTESIAN_POINT('Ctrl Pts',(2.82627835782077,1.14895307049812,1.10000025453558));
#14158=CARTESIAN_POINT('Ctrl Pts',(6.89526707210341,1.24931206297629,1.10000089539479));
#14159=CARTESIAN_POINT('Ctrl Pts',(10.9538643739116,1.56662321146826,1.09999817462385));
#14160=CARTESIAN_POINT('Ctrl Pts',(12.6856343728622,1.77018000694724,1.1));
#14161=CARTESIAN_POINT('Ctrl Pts',(0.500268515870817,1.1331394488043,1.0813211979534));
#14162=CARTESIAN_POINT('Ctrl Pts',(2.82529890252049,1.18902174635009,1.08130951558041));
#14163=CARTESIAN_POINT('Ctrl Pts',(6.89355973615254,1.28937215350496,1.08131090331441));
#14164=CARTESIAN_POINT('Ctrl Pts',(10.9502072694324,1.60665096558469,1.08120831497395));
#14165=CARTESIAN_POINT('Ctrl Pts',(12.6809355941985,1.8101648101409,1.08112518582372));
#14166=CARTESIAN_POINT('Ctrl Pts',(0.499889770519458,1.14890257814608,1.04159845594383));
#14167=CARTESIAN_POINT('Ctrl Pts',(2.82491374066927,1.20477605458053,1.04156824165266));
#14168=CARTESIAN_POINT('Ctrl Pts',(6.89288550108907,1.30512505153819,1.04157208085565));
#14169=CARTESIAN_POINT('Ctrl Pts',(10.948780858633,1.62227254848209,1.04130507279621));
#14170=CARTESIAN_POINT('Ctrl Pts',(12.6791127113589,1.82567684354491,1.04109086533338));
#14171=CARTESIAN_POINT('Ctrl Pts',(0.499867468633484,1.14983076779096,1.024283610038));
#14172=CARTESIAN_POINT('Ctrl Pts',(2.82489125498211,1.205696711939,1.02424794747454));
#14173=CARTESIAN_POINT('Ctrl Pts',(6.89284643152835,1.3060464758645,1.02425267669241));
#14174=CARTESIAN_POINT('Ctrl Pts',(10.9487000866048,1.62312515852299,1.02393618997858));
#14175=CARTESIAN_POINT('Ctrl Pts',(12.6790190612712,1.82647376985123,1.02368384096639));
#14176=CARTESIAN_POINT('Ctrl Pts',(12.6790190612712,1.82647376985123,1.02368384096639));
#14177=CARTESIAN_POINT('Ctrl Pts',(10.9487000866048,1.62312515852299,1.02393618997858));
#14178=CARTESIAN_POINT('Ctrl Pts',(6.89284643152835,1.3060464758645,1.02425267669241));
#14179=CARTESIAN_POINT('Ctrl Pts',(2.82489125498211,1.205696711939,1.02424794747454));
#14180=CARTESIAN_POINT('Ctrl Pts',(0.499867468633484,1.14983076779096,1.024283610038));
#14181=CARTESIAN_POINT('Ctrl Pts',(0.501786340877248,1.0699685826571,1.1));
#14182=CARTESIAN_POINT('Ctrl Pts',(2.82684356715236,1.12583341742443,1.1));
#14183=CARTESIAN_POINT('Ctrl Pts',(6.89625445951469,1.22619710828032,1.1));
#14184=CARTESIAN_POINT('Ctrl Pts',(10.9559704995293,1.54352620424957,1.1));
#14185=CARTESIAN_POINT('Ctrl Pts',(12.6883460378814,1.74710477827991,1.1));
#14186=CARTESIAN_POINT('Origin',(0.347167001354737,-1.15283299864526,0.9));
#14187=CARTESIAN_POINT('',(0.347167001354737,1.00658943961019,0.9));
#14188=CARTESIAN_POINT('Ctrl Pts',(0.347167001354737,1.00658943961019,0.9));
#14189=CARTESIAN_POINT('Ctrl Pts',(0.349336454155793,1.00442120424608,0.941395625434512));
#14190=CARTESIAN_POINT('Ctrl Pts',(0.351505906960267,1.0022529701308,0.982791250934257));
#14191=CARTESIAN_POINT('Ctrl Pts',(0.35367535976817,1.0000847372682,1.02418687649944));
#14192=CARTESIAN_POINT('',(0.347167001354737,-1.00658943961019,0.9));
#14193=CARTESIAN_POINT('',(0.347167001354737,-1.15283299864526,0.9));
#14194=CARTESIAN_POINT('Ctrl Pts',(0.353675359768457,-1.00008473726791,
1.02418687650491));
#14195=CARTESIAN_POINT('Ctrl Pts',(0.351505906960458,-1.0022529701306,0.982791250937906));
#14196=CARTESIAN_POINT('Ctrl Pts',(0.349336454155888,-1.00442120424599,
0.941395625436337));
#14197=CARTESIAN_POINT('Ctrl Pts',(0.347167001354737,-1.00658943961019,
0.900000000000001));
#14198=CARTESIAN_POINT('Ctrl Pts',(0.346996296805428,1.00676004836741,0.896742763161407));
#14199=CARTESIAN_POINT('Ctrl Pts',(0.349222651122738,1.0045349433512,0.939224134205317));
#14200=CARTESIAN_POINT('Ctrl Pts',(0.351449005443648,1.00230983965007,0.981705505317921));
#14201=CARTESIAN_POINT('Ctrl Pts',(0.35367535976817,1.0000847372682,1.02418687649944));
#14202=CARTESIAN_POINT('Ctrl Pts',(0.347116900426942,1.05081591929015,0.899044017348554));
#14203=CARTESIAN_POINT('Ctrl Pts',(0.349343263597644,1.04859056550012,0.941525373982715));
#14204=CARTESIAN_POINT('Ctrl Pts',(0.351569598045448,1.04636522758029,0.98400673296308));
#14205=CARTESIAN_POINT('Ctrl Pts',(0.353795961241832,1.04413987589222,1.02648808970312));
#14206=CARTESIAN_POINT('Ctrl Pts',(0.383592239441417,1.12715274970112,0.901130824661994));
#14207=CARTESIAN_POINT('Ctrl Pts',(0.38581816402279,1.12492699736917,0.943612181832344));
#14208=CARTESIAN_POINT('Ctrl Pts',(0.388044096297176,1.12270123909217,0.986093538279035));
#14209=CARTESIAN_POINT('Ctrl Pts',(0.390270019973987,1.12047548800691,1.02857489555427));
#14210=CARTESIAN_POINT('Ctrl Pts',(0.460164343209507,1.15561854687756,0.898608842835867));
#14211=CARTESIAN_POINT('Ctrl Pts',(0.462389604568499,1.15339312775892,0.941090251624243));
#14212=CARTESIAN_POINT('Ctrl Pts',(0.464614871986574,1.15116771740584,0.983571660556392));
#14213=CARTESIAN_POINT('Ctrl Pts',(0.466840131020026,1.14894230022584,1.02605306955844));
#14214=CARTESIAN_POINT('Ctrl Pts',(0.493196683694039,1.15650174777388,0.896923951850831));
#14215=CARTESIAN_POINT('Ctrl Pts',(0.49542175781822,1.15427660869429,0.939405385103827));
#14216=CARTESIAN_POINT('Ctrl Pts',(0.497646830577711,1.15205147087705,0.981886818489558));
#14217=CARTESIAN_POINT('Ctrl Pts',(0.499871901968125,1.1498263343261,1.02436825200844));
#14218=CARTESIAN_POINT('',(0.493357799610229,1.15634062715414,0.9));
#14219=CARTESIAN_POINT('Ctrl Pts',(0.499867468633513,1.14983076779054,1.02428361004581));
#14220=CARTESIAN_POINT('Ctrl Pts',(0.497697580259738,1.1520007197087,0.982855739904038));
#14221=CARTESIAN_POINT('Ctrl Pts',(0.495527690583954,1.15417067283112,0.941427869888898));
#14222=CARTESIAN_POINT('Ctrl Pts',(0.493357799610229,1.15634062715414,0.9));
#14223=CARTESIAN_POINT('Ctrl Pts',(0.493357799610229,1.15634062715414,0.9));
#14224=CARTESIAN_POINT('Ctrl Pts',(0.482602647031033,1.1560824793541,0.899999999999731));
#14225=CARTESIAN_POINT('Ctrl Pts',(0.471926867235344,1.1546337250523,0.899998382330426));
#14226=CARTESIAN_POINT('Ctrl Pts',(0.461511103461674,1.15208577142905,0.899997935562642));
#14227=CARTESIAN_POINT('Ctrl Pts',(0.453002267216956,1.15000429947842,0.899997570589511));
#14228=CARTESIAN_POINT('Ctrl Pts',(0.444666263429443,1.14718801542572,0.899997957558805));
#14229=CARTESIAN_POINT('Ctrl Pts',(0.436607964282466,1.14366186386534,0.899998978246166));
#14230=CARTESIAN_POINT('Ctrl Pts',(0.426757323168539,1.13935141908028,0.900000225956719));
#14231=CARTESIAN_POINT('Ctrl Pts',(0.417425277328103,1.13402704260718,0.900002535631972));
#14232=CARTESIAN_POINT('Ctrl Pts',(0.408793513884033,1.1277570068973,0.900002417864976));
#14233=CARTESIAN_POINT('Ctrl Pts',(0.406442206080559,1.1260490379535,0.900002385785035));
#14234=CARTESIAN_POINT('Ctrl Pts',(0.404142986411405,1.12427063023042,0.900002152965402));
#14235=CARTESIAN_POINT('Ctrl Pts',(0.40189988757483,1.12242258952304,0.900001599918915));
#14236=CARTESIAN_POINT('Ctrl Pts',(0.397433290854798,1.11874265691041,0.900000498658648));
#14237=CARTESIAN_POINT('Ctrl Pts',(0.393188994678067,1.11478677136369,0.899998147353889));
#14238=CARTESIAN_POINT('Ctrl Pts',(0.389180227688998,1.11057998277971,0.899995556820878));
#14239=CARTESIAN_POINT('Ctrl Pts',(0.381747711834384,1.10278032195316,0.899990753803459));
#14240=CARTESIAN_POINT('Ctrl Pts',(0.375201641992584,1.09420365251288,0.899985427555825));
#14241=CARTESIAN_POINT('Ctrl Pts',(0.369602030462105,1.08503231460429,0.899982994308828));
#14242=CARTESIAN_POINT('Ctrl Pts',(0.365103987453251,1.07766518348509,0.899981039735804));
#14243=CARTESIAN_POINT('Ctrl Pts',(0.361217082581294,1.06991300661492,0.899980859474918));
#14244=CARTESIAN_POINT('Ctrl Pts',(0.357992910300892,1.06185737523451,0.899982473761482));
#14245=CARTESIAN_POINT('Ctrl Pts',(0.354005020049728,1.0518935857546,0.899984470428251));
#14246=CARTESIAN_POINT('Ctrl Pts',(0.351071168910505,1.04156966067519,0.899989252895565));
#14247=CARTESIAN_POINT('Ctrl Pts',(0.349267161175031,1.03104850244781,0.899993624760896));
#14248=CARTESIAN_POINT('Ctrl Pts',(0.347885225415831,1.022988911296,0.899996973769283));
#14249=CARTESIAN_POINT('Ctrl Pts',(0.347167001481006,1.014812725533,0.899999999989923));
#14250=CARTESIAN_POINT('Ctrl Pts',(0.347167001354737,1.00658943961019,0.900000000000001));
#14251=CARTESIAN_POINT('Ctrl Pts',(0.493357799610229,1.15634062715414,0.9));
#14252=CARTESIAN_POINT('Ctrl Pts',(0.495478181125715,1.15416948447463,0.941427870236244));
#14253=CARTESIAN_POINT('Ctrl Pts',(0.4975985626412,1.15199834179512,0.982855740472488));
#14254=CARTESIAN_POINT('Ctrl Pts',(0.499718944156686,1.14982719911562,1.02428361070873));
#14255=CARTESIAN_POINT('Ctrl Pts',(4.55741138981048,1.2538870134557,0.9));
#14256=CARTESIAN_POINT('Ctrl Pts',(4.55812062853622,1.25171587077619,0.941427870236244));
#14257=CARTESIAN_POINT('Ctrl Pts',(4.55882986726197,1.24954472809669,0.982855740472489));
#14258=CARTESIAN_POINT('Ctrl Pts',(4.55953910598771,1.24737358541718,1.02428361070873));
#14259=CARTESIAN_POINT('Ctrl Pts',(8.62146498001072,1.3558778793304,0.9));
#14260=CARTESIAN_POINT('Ctrl Pts',(8.62076307594673,1.35370673665089,0.941427870236244));
#14261=CARTESIAN_POINT('Ctrl Pts',(8.62006117188274,1.35153559397139,0.982855740472488));
#14262=CARTESIAN_POINT('Ctrl Pts',(8.61935926781874,1.34936445129188,1.02428361070873));
#14263=CARTESIAN_POINT('Ctrl Pts',(12.685518570211,1.83297820604925,0.9));
#14264=CARTESIAN_POINT('Ctrl Pts',(12.6834055233572,1.83080706336974,0.941427870236244));
#14265=CARTESIAN_POINT('Ctrl Pts',(12.6812924765035,1.82863592069023,0.982855740472488));
#14266=CARTESIAN_POINT('Ctrl Pts',(12.6791794296498,1.82646477801072,1.02428361070873));
#14267=CARTESIAN_POINT('',(12.685518570211,1.83297820604925,0.9));
#14268=CARTESIAN_POINT('Ctrl Pts',(12.685518570211,1.83297820604925,0.9));
#14269=CARTESIAN_POINT('Ctrl Pts',(12.6833520729681,1.83081006895277,0.941227947697879));
#14270=CARTESIAN_POINT('Ctrl Pts',(12.6811855699938,1.8286419235626,0.982455894687412));
#14271=CARTESIAN_POINT('Ctrl Pts',(12.6790190612712,1.82647376985122,1.02368384096639));
#14272=CARTESIAN_POINT('Ctrl Pts',(0.493357799610229,1.15634062715414,0.9));
#14273=CARTESIAN_POINT('Ctrl Pts',(4.55741138981048,1.2538870134557,0.9));
#14274=CARTESIAN_POINT('Ctrl Pts',(8.62146498001073,1.3558778793304,0.9));
#14275=CARTESIAN_POINT('Ctrl Pts',(12.685518570211,1.83297820604925,0.9));
#14276=CARTESIAN_POINT('Ctrl Pts',(12.6857396223418,1.83319942548878,0.895793428058847));
#14277=CARTESIAN_POINT('Ctrl Pts',(12.6834994414517,1.83095754915284,0.938423566452776));
#14278=CARTESIAN_POINT('Ctrl Pts',(12.6812592544344,1.82871566395046,0.981053704089438));
#14279=CARTESIAN_POINT('Ctrl Pts',(12.6790190612712,1.82647376985122,1.02368384096639));
#14280=CARTESIAN_POINT('Ctrl Pts',(12.7096132738247,1.83593722009608,0.897188525535458));
#14281=CARTESIAN_POINT('Ctrl Pts',(12.7073735515623,1.83369637734113,0.939818742641338));
#14282=CARTESIAN_POINT('Ctrl Pts',(12.7051338254027,1.83145551796363,0.982448958687984));
#14283=CARTESIAN_POINT('Ctrl Pts',(12.7028940916787,1.82921465970329,1.02507917444001));
#14284=CARTESIAN_POINT('Ctrl Pts',(12.7586310095219,1.82964538228831,0.8994266592275));
#14285=CARTESIAN_POINT('Ctrl Pts',(12.7563927428119,1.82740607701793,0.942057032676437));
#14286=CARTESIAN_POINT('Ctrl Pts',(12.7541544559015,1.82516675428928,0.984687404166494));
#14287=CARTESIAN_POINT('Ctrl Pts',(12.7519161806021,1.82292743696394,1.02731777659207));
#14288=CARTESIAN_POINT('Ctrl Pts',(12.8300025526753,1.78023902864912,0.90056967297836));
#14289=CARTESIAN_POINT('Ctrl Pts',(12.8277672375473,1.7780001144899,0.943200215636435));
#14290=CARTESIAN_POINT('Ctrl Pts',(12.8255319263559,1.7757611919149,0.985830758073823));
#14291=CARTESIAN_POINT('Ctrl Pts',(12.8232966088089,1.77352226682369,1.02846130007111));
#14292=CARTESIAN_POINT('Ctrl Pts',(12.8529050075203,1.72043671272769,0.898625988813541));
#14293=CARTESIAN_POINT('Ctrl Pts',(12.8506708576607,1.71819639833573,0.941256511626846));
#14294=CARTESIAN_POINT('Ctrl Pts',(12.8484366444933,1.71595605563573,0.983887029620282));
#14295=CARTESIAN_POINT('Ctrl Pts',(12.8462024947189,1.71371572743615,1.0265175517275));
#14296=CARTESIAN_POINT('Ctrl Pts',(12.853004077605,1.68438049200639,0.896735618985435));
#14297=CARTESIAN_POINT('Ctrl Pts',(12.8507699092581,1.68213930602179,0.939366090596142));
#14298=CARTESIAN_POINT('Ctrl Pts',(12.8485357409326,1.67989811224666,0.981996561798403));
#14299=CARTESIAN_POINT('Ctrl Pts',(12.8463015726285,1.67765691065502,1.02462703259085));
#14300=CARTESIAN_POINT('',(12.8528329986453,1.6842088756636,0.9));
#14301=CARTESIAN_POINT('Ctrl Pts',(12.8463246402318,1.67768005087614,1.02418687649944));
#14302=CARTESIAN_POINT('Ctrl Pts',(12.8484940930161,1.67985633316752,0.982791251385616));
#14303=CARTESIAN_POINT('Ctrl Pts',(12.8506635458206,1.68203260808875,0.941395625885387));
#14304=CARTESIAN_POINT('Ctrl Pts',(12.8528329986453,1.6842088756636,0.9));
#14305=CARTESIAN_POINT('Ctrl Pts',(12.8528329986453,1.6842088756636,0.900000000000001));
#14306=CARTESIAN_POINT('Ctrl Pts',(12.8528329990894,1.69496116035511,0.900000000031321));
#14307=CARTESIAN_POINT('Ctrl Pts',(12.8516279916809,1.7056415234076,0.899996564780585));
#14308=CARTESIAN_POINT('Ctrl Pts',(12.8493173682463,1.71608623918215,0.899994054968391));
#14309=CARTESIAN_POINT('Ctrl Pts',(12.847426586744,1.72463314262321,0.89999200119087));
#14310=CARTESIAN_POINT('Ctrl Pts',(12.8447941883809,1.73302290492875,0.899990534206534));
#14311=CARTESIAN_POINT('Ctrl Pts',(12.8414494901174,1.74115996769839,0.899990418365756));
#14312=CARTESIAN_POINT('Ctrl Pts',(12.8373567881217,1.75111679202539,0.899990276618506));
#14313=CARTESIAN_POINT('Ctrl Pts',(12.8322422209112,1.76059035368083,0.899992293328656));
#14314=CARTESIAN_POINT('Ctrl Pts',(12.8261823199623,1.76941466903515,0.899994578235276));
#14315=CARTESIAN_POINT('Ctrl Pts',(12.8228443945912,1.77427529404419,0.899995836811587));
#14316=CARTESIAN_POINT('Ctrl Pts',(12.819218773978,1.77893868154471,0.899997117508201));
#14317=CARTESIAN_POINT('Ctrl Pts',(12.8153125401773,1.78337342370743,0.899997612422461));
#14318=CARTESIAN_POINT('Ctrl Pts',(12.8134661485928,1.78546962967624,0.899997846357645));
#14319=CARTESIAN_POINT('Ctrl Pts',(12.8115570049875,1.7875146981109,0.899997899028016));
#14320=CARTESIAN_POINT('Ctrl Pts',(12.8095877759185,1.78950657520057,0.899997852068527));
#14321=CARTESIAN_POINT('Ctrl Pts',(12.802037518393,1.7971436679198,0.899997672020282));
#14322=CARTESIAN_POINT('Ctrl Pts',(12.7936869960543,1.80392089040634,0.899996345477631));
#14323=CARTESIAN_POINT('Ctrl Pts',(12.7847141304683,1.80975200096328,0.89999606036814));
#14324=CARTESIAN_POINT('Ctrl Pts',(12.7774211187199,1.81449144093269,0.899995828635385));
#14325=CARTESIAN_POINT('Ctrl Pts',(12.7697156358622,1.81860556854039,0.899996199361957));
#14326=CARTESIAN_POINT('Ctrl Pts',(12.761679297021,1.82202698480181,0.89999650903244));
#14327=CARTESIAN_POINT('Ctrl Pts',(12.7599722005109,1.82275376945776,0.899996574813315));
#14328=CARTESIAN_POINT('Ctrl Pts',(12.7582527406357,1.82344811243542,0.899996631272027));
#14329=CARTESIAN_POINT('Ctrl Pts',(12.7565217796305,1.82410952822173,0.899996662852262));
#14330=CARTESIAN_POINT('Ctrl Pts',(12.7461353325744,1.82807828316523,0.899996852346099));
#14331=CARTESIAN_POINT('Ctrl Pts',(12.7353361797362,1.83086624339127,0.899996468077086));
#14332=CARTESIAN_POINT('Ctrl Pts',(12.7243231747362,1.83245001845531,0.899997092905297));
#14333=CARTESIAN_POINT('Ctrl Pts',(12.713718016754,1.83397514123175,0.899997694594108));
#14334=CARTESIAN_POINT('Ctrl Pts',(12.702988146695,1.83437268605832,0.899999174299692));
#14335=CARTESIAN_POINT('Ctrl Pts',(12.6923097158784,1.83361665751845,0.899999788491474));
#14336=CARTESIAN_POINT('Ctrl Pts',(12.6900431251392,1.83345618381998,0.899999918859074));
#14337=CARTESIAN_POINT('Ctrl Pts',(12.6877788433122,1.83324355125563,0.900000000001074));
#14338=CARTESIAN_POINT('Ctrl Pts',(12.685518570211,1.83297820604925,0.9));
#14339=CARTESIAN_POINT('Origin',(6.88201982834292,-2.22044604925031E-16,
1.1));
#14340=CARTESIAN_POINT('Origin',(12.8528329986453,1.85283299864526,0.9));
#14341=CARTESIAN_POINT('',(12.8528329986453,-1.6842088756636,0.9));
#14342=CARTESIAN_POINT('Ctrl Pts',(12.8528329986453,-1.6842088756636,0.9));
#14343=CARTESIAN_POINT('Ctrl Pts',(12.8506635458206,-1.68203260808875,0.941395625885387));
#14344=CARTESIAN_POINT('Ctrl Pts',(12.8484940930161,-1.67985633316752,0.982791251385615));
#14345=CARTESIAN_POINT('Ctrl Pts',(12.8463246402318,-1.67768005087614,1.02418687649944));
#14346=CARTESIAN_POINT('',(12.8528329986453,1.85283299864526,0.9));
#14347=CARTESIAN_POINT('Ctrl Pts',(0.49319751180194,-1.1565009196418,0.896939762205254));
#14348=CARTESIAN_POINT('Ctrl Pts',(0.495422309889911,-1.15427605660646,
0.939415925341967));
#14349=CARTESIAN_POINT('Ctrl Pts',(0.49764710661353,-1.15205119483315,0.981892088611382));
#14350=CARTESIAN_POINT('Ctrl Pts',(0.499871901968411,-1.14982633432581,
1.02436825201392));
#14351=CARTESIAN_POINT('Ctrl Pts',(0.449154391250001,-1.15532331830903,
0.899186283506502));
#14352=CARTESIAN_POINT('Ctrl Pts',(0.451379443529967,-1.1530980743259,0.94166241338335));
#14353=CARTESIAN_POINT('Ctrl Pts',(0.453604490603533,-1.15087286444957,
0.984138545342204));
#14354=CARTESIAN_POINT('Ctrl Pts',(0.45582954070428,-1.14864762219213,1.02661467541392));
#14355=CARTESIAN_POINT('Ctrl Pts',(0.373709798968055,-1.1170292567097,0.901134386478875));
#14356=CARTESIAN_POINT('Ctrl Pts',(0.37593556973194,-1.11480381901192,0.943610469359475));
#14357=CARTESIAN_POINT('Ctrl Pts',(0.378161343437362,-1.11257837175868,
0.98608655157339));
#14358=CARTESIAN_POINT('Ctrl Pts',(0.380387113556173,-1.11035293539114,
1.02856263455032));
#14359=CARTESIAN_POINT('Ctrl Pts',(0.347087578105715,-1.039801123372,0.898484514129229));
#14360=CARTESIAN_POINT('Ctrl Pts',(0.349313658773859,-1.03757611304936,
0.940960604750146));
#14361=CARTESIAN_POINT('Ctrl Pts',(0.351539730193144,-1.03535109931323,
0.983436695671939));
#14362=CARTESIAN_POINT('Ctrl Pts',(0.353765810873703,-1.03312609123593,
1.02591278640767));
#14363=CARTESIAN_POINT('Ctrl Pts',(0.346997125389779,-1.00675922024802,
0.896758573492677));
#14364=CARTESIAN_POINT('Ctrl Pts',(0.349223203512402,-1.00453439127183,
0.939234674428006));
#14365=CARTESIAN_POINT('Ctrl Pts',(0.351449281638624,-1.0023095636104,0.98171077543201));
#14366=CARTESIAN_POINT('Ctrl Pts',(0.353675359768457,-1.00008473726791,
1.02418687650491));
#14367=CARTESIAN_POINT('',(0.493357799610228,-1.15634062715414,0.9));
#14368=CARTESIAN_POINT('Ctrl Pts',(0.347167001354737,-1.00658943961019,
0.900000000000001));
#14369=CARTESIAN_POINT('Ctrl Pts',(0.347167001425373,-1.01734828759763,
0.899999999998142));
#14370=CARTESIAN_POINT('Ctrl Pts',(0.348359077578701,-1.02805639415283,
0.899998433630397));
#14371=CARTESIAN_POINT('Ctrl Pts',(0.350656214310366,-1.0385309656087,0.899998024549738));
#14372=CARTESIAN_POINT('Ctrl Pts',(0.352533324612331,-1.04709028457193,
0.899997690268584));
#14373=CARTESIAN_POINT('Ctrl Pts',(0.355149562279486,-1.05549438497634,
0.899998101733499));
#14374=CARTESIAN_POINT('Ctrl Pts',(0.358482507184576,-1.0636377229308,0.899999127793999));
#14375=CARTESIAN_POINT('Ctrl Pts',(0.362555301547827,-1.07358872478153,
0.900000381620131));
#14376=CARTESIAN_POINT('Ctrl Pts',(0.367654000430903,-1.08304569392442,
0.900002668831236));
#14377=CARTESIAN_POINT('Ctrl Pts',(0.373714802804109,-1.09182534802447,
0.900002509451715));
#14378=CARTESIAN_POINT('Ctrl Pts',(0.375364773372187,-1.09421548879643,
0.90000246606282));
#14379=CARTESIAN_POINT('Ctrl Pts',(0.377086318771695,-1.09655531312597,
0.900002220932131));
#14380=CARTESIAN_POINT('Ctrl Pts',(0.378878733123435,-1.0988407769929,0.900001655250762));
#14381=CARTESIAN_POINT('Ctrl Pts',(0.382452759797804,-1.10339793132263,
0.900000527297116));
#14382=CARTESIAN_POINT('Ctrl Pts',(0.386308400219556,-1.10773917492176,
0.899998144709029));
#14383=CARTESIAN_POINT('Ctrl Pts',(0.390420886280218,-1.11185064093822,
0.899995523300098));
#14384=CARTESIAN_POINT('Ctrl Pts',(0.398040323803163,-1.11946818856709,
0.899990666466232));
#14385=CARTESIAN_POINT('Ctrl Pts',(0.406457812610252,-1.12621813960646,
0.899985292057237));
#14386=CARTESIAN_POINT('Ctrl Pts',(0.41549254786509,-1.13203603704298,0.899982834497606));
#14387=CARTESIAN_POINT('Ctrl Pts',(0.422749169000726,-1.13670892189372,
0.899980860606988));
#14388=CARTESIAN_POINT('Ctrl Pts',(0.430405328105449,-1.14078012415116,
0.899980677151631));
#14389=CARTESIAN_POINT('Ctrl Pts',(0.438380728308649,-1.14419607025517,
0.899982305341352));
#14390=CARTESIAN_POINT('Ctrl Pts',(0.448245442291908,-1.14842122892304,
0.899984319237269));
#14391=CARTESIAN_POINT('Ctrl Pts',(0.458495412124849,-1.1516012547891,0.899989147510445));
#14392=CARTESIAN_POINT('Ctrl Pts',(0.468969635281765,-1.1536564168707,0.899993562691215));
#14393=CARTESIAN_POINT('Ctrl Pts',(0.476989372009021,-1.15522998071208,
0.899996943236659));
#14394=CARTESIAN_POINT('Ctrl Pts',(0.485141446557615,-1.15614341614473,
0.89999999999177));
#14395=CARTESIAN_POINT('Ctrl Pts',(0.493357799610229,-1.15634062715414,
0.9));
#14396=CARTESIAN_POINT('Ctrl Pts',(0.493357799610229,-1.15634062715414,
0.9));
#14397=CARTESIAN_POINT('Ctrl Pts',(0.495527690583772,-1.1541706728313,0.941427869885423));
#14398=CARTESIAN_POINT('Ctrl Pts',(0.497697580259374,-1.15200071970906,
0.982855739897088));
#14399=CARTESIAN_POINT('Ctrl Pts',(0.499867468632967,-1.14983076779109,
1.02428361003538));
#14400=CARTESIAN_POINT('Ctrl Pts',(12.8530083952718,-1.68438482323521,0.896653232994753));
#14401=CARTESIAN_POINT('Ctrl Pts',(12.8507727877026,-1.68214219351771,0.939311166602882));
#14402=CARTESIAN_POINT('Ctrl Pts',(12.8485371801548,-1.67989955599965,0.98196909980204));
#14403=CARTESIAN_POINT('Ctrl Pts',(12.8463015726285,-1.67765691065502,1.02462703259086));
#14404=CARTESIAN_POINT('Ctrl Pts',(12.852942348552,-1.70842230260233,0.897913479482771));
#14405=CARTESIAN_POINT('Ctrl Pts',(12.8507067417858,-1.70618025058462,0.940571446443912));
#14406=CARTESIAN_POINT('Ctrl Pts',(12.8484711274102,-1.70393818829512,0.983229412467123));
#14407=CARTESIAN_POINT('Ctrl Pts',(12.8462355206888,-1.70169612184244,1.02588737868196));
#14408=CARTESIAN_POINT('Ctrl Pts',(12.8409786353997,-1.75638702494578,0.899808108153313));
#14409=CARTESIAN_POINT('Ctrl Pts',(12.838742445636,-1.75414612041198,0.942466110756886));
#14410=CARTESIAN_POINT('Ctrl Pts',(12.8365062537503,-1.75190518941781,0.985124111849326));
#14411=CARTESIAN_POINT('Ctrl Pts',(12.8342700627828,-1.74966427281549,1.02778211378599));
#14412=CARTESIAN_POINT('Ctrl Pts',(12.7836010260412,-1.82153168011476,0.900225885582409));
#14413=CARTESIAN_POINT('Ctrl Pts',(12.7813622549889,-1.8192914414386,0.942883795866658));
#14414=CARTESIAN_POINT('Ctrl Pts',(12.7791234760524,-1.81705120036295,0.985541705643422));
#14415=CARTESIAN_POINT('Ctrl Pts',(12.7768846983302,-1.81481095080325,1.02819961506361));
#14416=CARTESIAN_POINT('Ctrl Pts',(12.7215544275214,-1.83731044697508,0.89780368869924));
#14417=CARTESIAN_POINT('Ctrl Pts',(12.7193134882941,-1.83506869652207,0.940461407834127));
#14418=CARTESIAN_POINT('Ctrl Pts',(12.7170725571902,-1.83282686943458,0.983119123314088));
#14419=CARTESIAN_POINT('Ctrl Pts',(12.7148316068824,-1.83058510462933,1.02577684117682));
#14420=CARTESIAN_POINT('Ctrl Pts',(12.6857439516282,-1.83320375805174,0.895711042712126));
#14421=CARTESIAN_POINT('Ctrl Pts',(12.6835023276506,-1.83096043753957,0.938368642889274));
#14422=CARTESIAN_POINT('Ctrl Pts',(12.6812606975378,-1.82871710814956,0.981026242308181));
#14423=CARTESIAN_POINT('Ctrl Pts',(12.6790190612712,-1.82647376985122,1.02368384096639));
#14424=CARTESIAN_POINT('',(12.685518570211,-1.83297820604925,0.9));
#14425=CARTESIAN_POINT('Ctrl Pts',(12.6790190612712,-1.82647376985122,1.02368384096639));
#14426=CARTESIAN_POINT('Ctrl Pts',(12.6811855699938,-1.8286419235626,0.982455894687418));
#14427=CARTESIAN_POINT('Ctrl Pts',(12.6833520729681,-1.83081006895277,0.941227947697881));
#14428=CARTESIAN_POINT('Ctrl Pts',(12.685518570211,-1.83297820604925,0.9));
#14429=CARTESIAN_POINT('Ctrl Pts',(12.685518570211,-1.83297820604925,0.9));
#14430=CARTESIAN_POINT('Ctrl Pts',(12.6962007718831,-1.83423224573831,0.900000000027109));
#14431=CARTESIAN_POINT('Ctrl Pts',(12.7069522081469,-1.8342814865544,0.899996797888993));
#14432=CARTESIAN_POINT('Ctrl Pts',(12.7175986228217,-1.83320546389923,0.899994443686255));
#14433=CARTESIAN_POINT('Ctrl Pts',(12.7263221437181,-1.83232378622612,0.899992514685985));
#14434=CARTESIAN_POINT('Ctrl Pts',(12.7349759538105,-1.83068541925521,0.899991134073322));
#14435=CARTESIAN_POINT('Ctrl Pts',(12.7434612806603,-1.82830833949467,0.899991022249493));
#14436=CARTESIAN_POINT('Ctrl Pts',(12.7538268490808,-1.82540452879472,0.899990885646912));
#14437=CARTESIAN_POINT('Ctrl Pts',(12.7638319405548,-1.82143037312377,0.899992779825431));
#14438=CARTESIAN_POINT('Ctrl Pts',(12.7733027638617,-1.81644210162737,0.899994914291513));
#14439=CARTESIAN_POINT('Ctrl Pts',(12.7785122133597,-1.81369829070399,0.899996088359796));
#14440=CARTESIAN_POINT('Ctrl Pts',(12.7835598637901,-1.81064675361041,0.899997279965736));
#14441=CARTESIAN_POINT('Ctrl Pts',(12.7884138119185,-1.80729078554336,0.899997716205233));
#14442=CARTESIAN_POINT('Ctrl Pts',(12.7907292666901,-1.80568990476168,0.899997924302393));
#14443=CARTESIAN_POINT('Ctrl Pts',(12.7930005978609,-1.80401968744988,0.8999979548189));
#14444=CARTESIAN_POINT('Ctrl Pts',(12.7952253950699,-1.80228259226775,0.89999788947913));
#14445=CARTESIAN_POINT('Ctrl Pts',(12.8036908359575,-1.7956728767752,0.899997640858734));
#14446=CARTESIAN_POINT('Ctrl Pts',(12.8113954895597,-1.78816822909976,0.899996334032805));
#14447=CARTESIAN_POINT('Ctrl Pts',(12.818232559256,-1.77993499666286,0.899996088064289));
#14448=CARTESIAN_POINT('Ctrl Pts',(12.8237887404903,-1.77324421631459,0.899995888176659));
#14449=CARTESIAN_POINT('Ctrl Pts',(12.8287718252447,-1.76607091125846,0.899996310183797));
#14450=CARTESIAN_POINT('Ctrl Pts',(12.8331051219922,-1.75848815553817,0.899996624147351));
#14451=CARTESIAN_POINT('Ctrl Pts',(12.8340140186356,-1.75689769413573,0.899996690000312));
#14452=CARTESIAN_POINT('Ctrl Pts',(12.8348928881302,-1.75529157361675,0.899996744625968));
#14453=CARTESIAN_POINT('Ctrl Pts',(12.8357411680586,-1.75367056321155,0.89999677208873));
#14454=CARTESIAN_POINT('Ctrl Pts',(12.8409005734958,-1.74381125896804,0.89999693912265));
#14455=CARTESIAN_POINT('Ctrl Pts',(12.8449329422938,-1.7334030651393,0.899996442311536));
#14456=CARTESIAN_POINT('Ctrl Pts',(12.8477914282597,-1.72264121193733,0.899997037599541));
#14457=CARTESIAN_POINT('Ctrl Pts',(12.850541038206,-1.71228926375309,0.899997610213799));
#14458=CARTESIAN_POINT('Ctrl Pts',(12.8521849869391,-1.70168212150629,0.899999138466857));
#14459=CARTESIAN_POINT('Ctrl Pts',(12.8526768248801,-1.69099162083728,0.899999779783946));
#14460=CARTESIAN_POINT('Ctrl Pts',(12.8527806949164,-1.68873392048611,0.899999915222113));
#14461=CARTESIAN_POINT('Ctrl Pts',(12.8528329986625,-1.68647247255235,0.90000000000128));
#14462=CARTESIAN_POINT('Ctrl Pts',(12.8528329986453,-1.6842088756636,0.9));
#14463=CARTESIAN_POINT('Origin',(6.88173176806555,0.,0.9));
#14464=CARTESIAN_POINT('Ctrl Pts',(12.685518570211,-1.83297820604925,0.9));
#14465=CARTESIAN_POINT('Ctrl Pts',(8.62146498001073,-1.3558778793304,0.9));
#14466=CARTESIAN_POINT('Ctrl Pts',(4.55741138981048,-1.2538870134557,0.9));
#14467=CARTESIAN_POINT('Ctrl Pts',(0.493357799610228,-1.15634062715414,
0.9));
#14468=CARTESIAN_POINT('Ctrl Pts',(12.685518570211,-1.83297820604925,0.9));
#14469=CARTESIAN_POINT('Ctrl Pts',(12.6834055233574,-1.83080706336992,0.941427870232769));
#14470=CARTESIAN_POINT('Ctrl Pts',(12.6812924765039,-1.8286359206906,0.982855740465538));
#14471=CARTESIAN_POINT('Ctrl Pts',(12.6791794296503,-1.82646477801127,1.02428361069831));
#14472=CARTESIAN_POINT('Ctrl Pts',(8.62146498001072,-1.3558778793304,0.9));
#14473=CARTESIAN_POINT('Ctrl Pts',(8.62076307594679,-1.35370673665108,0.941427870232769));
#14474=CARTESIAN_POINT('Ctrl Pts',(8.62006117188285,-1.35153559397175,0.982855740465538));
#14475=CARTESIAN_POINT('Ctrl Pts',(8.61935926781891,-1.34936445129242,1.02428361069831));
#14476=CARTESIAN_POINT('Ctrl Pts',(4.55741138981048,-1.2538870134557,0.9));
#14477=CARTESIAN_POINT('Ctrl Pts',(4.55812062853616,-1.25171587077637,0.941427870232769));
#14478=CARTESIAN_POINT('Ctrl Pts',(4.55882986726185,-1.24954472809705,0.982855740465538));
#14479=CARTESIAN_POINT('Ctrl Pts',(4.55953910598754,-1.24737358541772,1.02428361069831));
#14480=CARTESIAN_POINT('Ctrl Pts',(0.493357799610228,-1.15634062715414,
0.9));
#14481=CARTESIAN_POINT('Ctrl Pts',(0.495478181125536,-1.15416948447481,
0.941427870232769));
#14482=CARTESIAN_POINT('Ctrl Pts',(0.497598562640844,-1.15199834179549,
0.982855740465538));
#14483=CARTESIAN_POINT('Ctrl Pts',(0.499718944156152,-1.14982719911616,
1.02428361069831));
#19601=UNCERTAINTY_MEASURE_WITH_UNIT(LENGTH_MEASURE(0.001),#19619,
'DISTANCE_ACCURACY_VALUE',
'Maximum model space distance between geometric entities at asserted c
onnectivities');
#19605=UNCERTAINTY_MEASURE_WITH_UNIT(LENGTH_MEASURE(0.001),#19619,
'DISTANCE_ACCURACY_VALUE',
'Maximum model space distance between geometric entities at asserted c
onnectivities');
#19614=(
GEOMETRIC_REPRESENTATION_CONTEXT(3)
GLOBAL_UNCERTAINTY_ASSIGNED_CONTEXT((#19601))
GLOBAL_UNIT_ASSIGNED_CONTEXT((#19619,#19621,#19622))
REPRESENTATION_CONTEXT('','3D')
);
#19618=(
GEOMETRIC_REPRESENTATION_CONTEXT(3)
GLOBAL_UNCERTAINTY_ASSIGNED_CONTEXT((#19605))
GLOBAL_UNIT_ASSIGNED_CONTEXT((#19619,#19621,#19622))
REPRESENTATION_CONTEXT('','3D')
);
#19619=(
LENGTH_UNIT()
NAMED_UNIT(*)
SI_UNIT(.CENTI.,.METRE.)
);
#19621=(
NAMED_UNIT(*)
PLANE_ANGLE_UNIT()
SI_UNIT($,.RADIAN.)
);
#19622=(
NAMED_UNIT(*)
SI_UNIT($,.STERADIAN.)
SOLID_ANGLE_UNIT()
);
#19631=SHAPE_DEFINITION_REPRESENTATION(#19643,#19671);
#19643=PRODUCT_DEFINITION_SHAPE('',$,#19684);
#19671=SHAPE_REPRESENTATION('',(#7583),#19614);
#19675=PRODUCT_DEFINITION_CONTEXT('part definition',#19713,'design');
#19684=PRODUCT_DEFINITION('2026-11-10-01-34-59-964','Soft grip layer',#19696,
#19675);
#19696=PRODUCT_DEFINITION_FORMATION('',$,#19723);
#19713=APPLICATION_CONTEXT(
'Core Data for Automotive Mechanical Design Process');
#19714=PRODUCT_CONTEXT('part definition',#19713,'mechanical');
#19723=PRODUCT('2026-11-10-01-34-59-964','Soft grip layer',$,(#19714));
#19732=PRESENTATION_STYLE_ASSIGNMENT((#19740));
#19740=SURFACE_STYLE_USAGE(.BOTH.,#19748);
#19748=SURFACE_SIDE_STYLE('',(#19756));
#19756=SURFACE_STYLE_FILL_AREA(#19764);
#19764=FILL_AREA_STYLE('Sky blue soft grip',(#19772));
#19772=FILL_AREA_STYLE_COLOUR('Sky blue soft grip',#19780);
#19780=COLOUR_RGB('Sky blue soft grip',0.27843137254902,0.309803921568627,
0.352941176470588);
ENDSEC;
END-ISO-10303-21;
